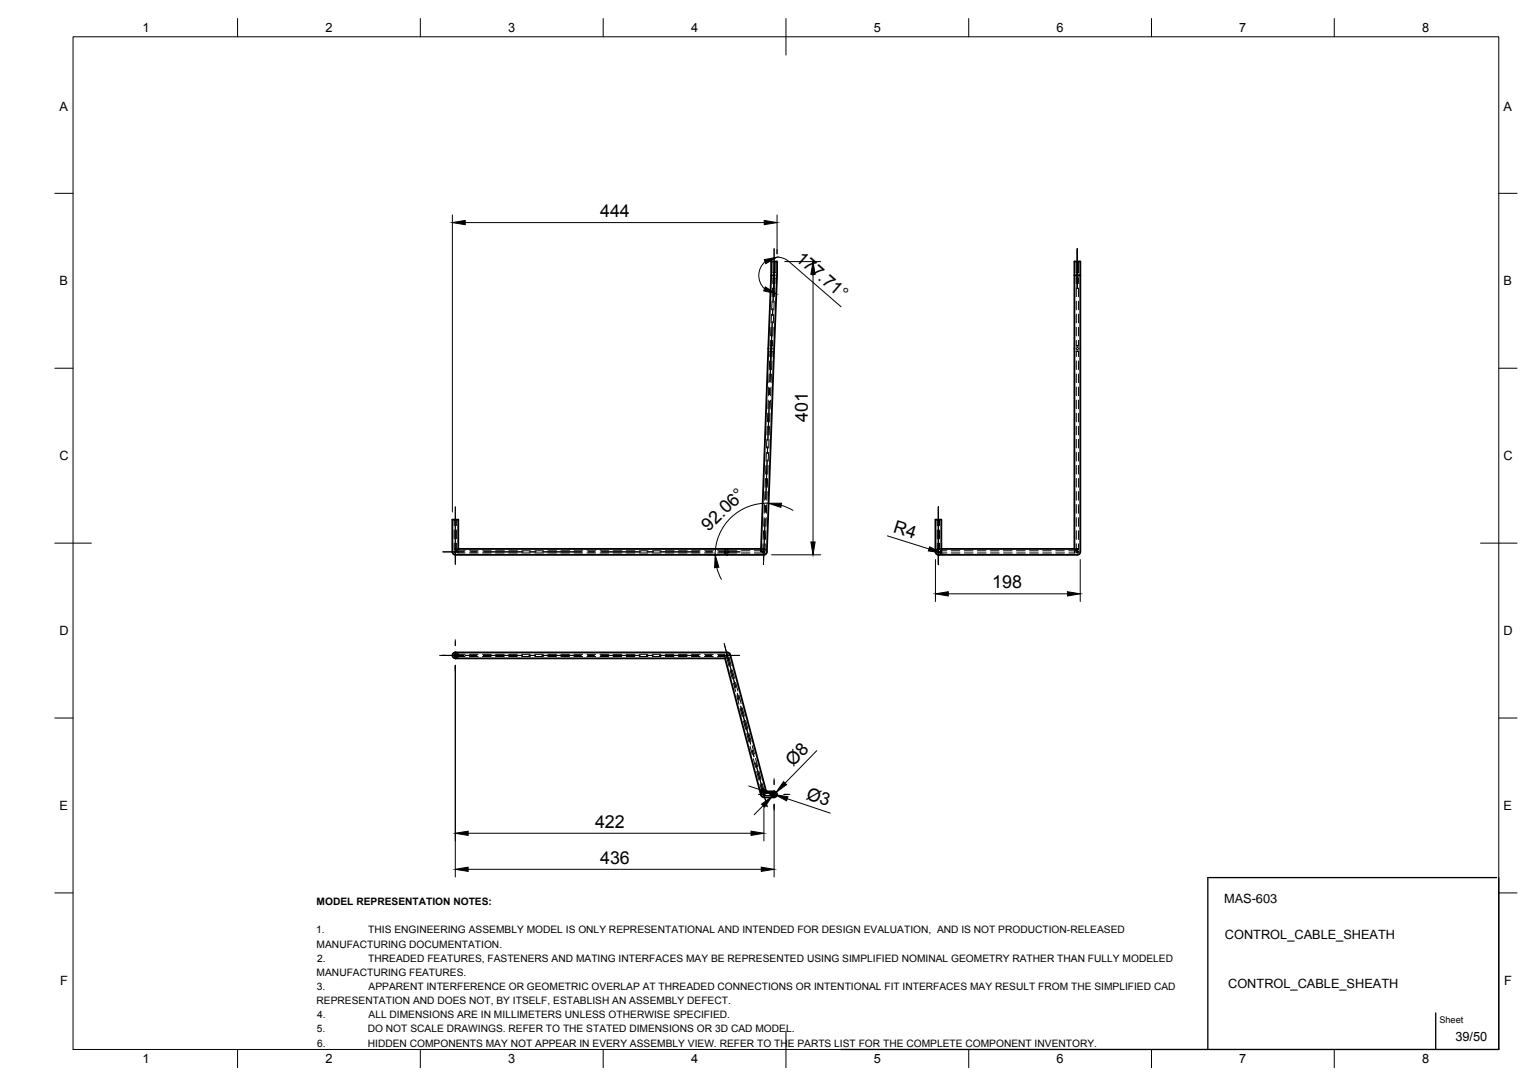
ISO-10303-21;
HEADER;
FILE_DESCRIPTION((''),'2;1');
FILE_NAME('CONTROL_CABLE_SHEATH.step','2026-10-01T22:06:14-07:00',(''),(''),'','','');
FILE_SCHEMA (('AUTOMOTIVE_DESIGN { 1 0 10303 214 3 1 1 }'));
ENDSEC;
DATA;
#10=MECHANICAL_DESIGN_GEOMETRIC_PRESENTATION_REPRESENTATION('',(#1012),#50440);
#21=B_SPLINE_CURVE_WITH_KNOTS('',3,(#47253,#47254,#47255,#47256,#47257,
#47258,#47259,#47260,#47261,#47262),.UNSPECIFIED.,.F.,.F.,(4,2,2,2,4),(0.22845269137107,
0.285543988105223,0.342635284839377,0.399770333790758,0.45690538274214),
 .UNSPECIFIED.) ;
#22=B_SPLINE_CURVE_WITH_KNOTS('',3,(#47263,#47264,#47265,#47266,#47267,
#47268,#47269,#47270,#47271,#47272),.UNSPECIFIED.,.F.,.F.,(4,2,2,2,4),(0.,
0.0571350489513819,0.114270097902764,0.171361394636917,0.22845269137107),
 .UNSPECIFIED.) ;
#23=B_SPLINE_CURVE_WITH_KNOTS('',3,(#47334,#47335,#47336,#47337,#47338,
#47339,#47340,#47341,#47342,#47343,#47344,#47345,#47346,#47347,#47348,#47349,
#47350,#47351),.UNSPECIFIED.,.F.,.F.,(4,2,2,2,2,2,2,2,4),(-0.453190854157869,
-0.399487512163789,-0.342402977588613,-0.285344500479048,-0.228286023369483,
-0.171227546259919,-0.114169069150354,-0.0570845345751771,-0.00338119258109968),
 .UNSPECIFIED.) ;
#24=B_SPLINE_CURVE_WITH_KNOTS('',3,(#47365,#47366,#47367,#47368,#47369,
#47370,#47371,#47372,#47373,#47374,#47375,#47376,#47377,#47378),
 .UNSPECIFIED.,.F.,.F.,(4,2,2,2,2,2,4),(0.577610065542725,0.589037524605606,
0.645581544002731,0.702125563399856,0.758669582796981,0.815213602194107,
0.826641061257004),.UNSPECIFIED.) ;
#25=B_SPLINE_CURVE_WITH_KNOTS('',3,(#47382,#47383,#47384,#47385,#47386,
#47387,#47388,#47389,#47390,#47391,#47392,#47393,#47394,#47395,#47396,#47397,
#47398,#47399),.UNSPECIFIED.,.F.,.F.,(4,2,2,2,2,2,2,2,4),(0.00338117995301888,
0.0570585291380164,0.114117058276033,0.171201519148796,0.228285980021559,
0.285370440894324,0.342454901767089,0.399513430905107,0.453190780090104),
 .UNSPECIFIED.) ;
#26=B_SPLINE_CURVE_WITH_KNOTS('',3,(#47419,#47420,#47421,#47422,#47423,
#47424,#47425,#47426,#47427,#47428,#47429,#47430,#47431,#47432,#47433,#47434,
#47435,#47436),.UNSPECIFIED.,.F.,.F.,(4,2,2,2,2,2,2,2,4),(-0.456905382742139,
-0.399770333790757,-0.342635284839376,-0.285543988105223,-0.228452691371069,
-0.171361394636916,-0.114270097902762,-0.0571350489513811,0.),
 .UNSPECIFIED.) ;
#27=B_SPLINE_CURVE_WITH_KNOTS('',3,(#47442,#47443,#47444,#47445,#47446,
#47447,#47448,#47449,#47450,#47451,#47452,#47453,#47454,#47455),
 .UNSPECIFIED.,.F.,.F.,(4,2,2,2,2,2,4),(0.102836390905491,0.113768884994942,
0.170566995159794,0.227365105324647,0.2841632154895,0.340961325654353,0.351893819743812),
 .UNSPECIFIED.) ;
#68=ORIENTED_CLOSED_SHELL('',*,#28679,.F.) ;
#69=ORIENTED_CLOSED_SHELL('',*,#28680,.F.) ;
#70=ORIENTED_CLOSED_SHELL('',*,#28681,.F.) ;
#71=ORIENTED_CLOSED_SHELL('',*,#28682,.F.) ;
#72=ORIENTED_CLOSED_SHELL('',*,#28684,.F.) ;
#73=ORIENTED_CLOSED_SHELL('',*,#28685,.F.) ;
#74=ORIENTED_CLOSED_SHELL('',*,#28686,.F.) ;
#75=ORIENTED_CLOSED_SHELL('',*,#28687,.F.) ;
#76=ORIENTED_CLOSED_SHELL('',*,#28688,.F.) ;
#80=BREP_WITH_VOIDS('CONTROL_CABLE_SHEATH',#28683,(#68,#69,#70,#71,#72,
#73,#74,#75,#76)) ;
#405=ELLIPSE('',#30976,0.400079928078316,0.4) ;
#406=ELLIPSE('',#30978,0.400079928078316,0.4) ;
#407=ELLIPSE('',#30982,0.400000809214436,0.4) ;
#408=ELLIPSE('',#30983,0.400000809214436,0.4) ;
#409=ELLIPSE('',#30986,0.563115453389195,0.4) ;
#410=ELLIPSE('',#30989,0.505057490139689,0.4) ;
#411=ELLIPSE('',#30992,0.565685424949243,0.4) ;
#412=ELLIPSE('',#30993,0.565685424949243,0.4) ;
#728=SPHERICAL_SURFACE('',#30943,0.15) ;
#729=SPHERICAL_SURFACE('',#30945,0.15) ;
#730=SPHERICAL_SURFACE('',#30947,0.15) ;
#731=SPHERICAL_SURFACE('',#30949,0.4) ;
#732=SPHERICAL_SURFACE('',#30953,0.4) ;
#733=SPHERICAL_SURFACE('',#30954,0.4) ;
#734=SPHERICAL_SURFACE('',#30957,0.4) ;
#735=SPHERICAL_SURFACE('',#30962,0.4) ;
#736=SPHERICAL_SURFACE('',#30965,0.4) ;
#737=SPHERICAL_SURFACE('',#30998,0.4) ;
#738=SPHERICAL_SURFACE('',#30999,0.4) ;
#739=SPHERICAL_SURFACE('',#31000,0.4) ;
#740=SPHERICAL_SURFACE('',#31001,0.4) ;
#741=SPHERICAL_SURFACE('',#31003,0.4) ;
#742=SPHERICAL_SURFACE('',#31009,0.15) ;
#743=SPHERICAL_SURFACE('',#31011,0.4) ;
#744=SPHERICAL_SURFACE('',#31021,0.4) ;
#745=SPHERICAL_SURFACE('',#31022,0.4) ;
#746=SPHERICAL_SURFACE('',#31033,0.4) ;
#747=SPHERICAL_SURFACE('',#31034,0.15) ;
#919=SHAPE_REPRESENTATION_RELATIONSHIP('SRR','None',#50652,#964) ;
#964=ADVANCED_BREP_SHAPE_REPRESENTATION('',(#80),#50421) ;
#1012=STYLED_ITEM('',(#50888),#80) ;
#1377=FACE_BOUND('',#5253,.T.) ;
#1378=FACE_BOUND('',#5261,.T.) ;
#2232=PLANE('',#30979) ;
#2233=PLANE('',#30997) ;
#3420=FACE_OUTER_BOUND('',#5239,.T.) ;
#3421=FACE_OUTER_BOUND('',#5240,.T.) ;
#3422=FACE_OUTER_BOUND('',#5241,.T.) ;
#3423=FACE_OUTER_BOUND('',#5242,.T.) ;
#3424=FACE_OUTER_BOUND('',#5243,.T.) ;
#3425=FACE_OUTER_BOUND('',#5244,.T.) ;
#3426=FACE_OUTER_BOUND('',#5245,.T.) ;
#3427=FACE_OUTER_BOUND('',#5246,.T.) ;
#3428=FACE_OUTER_BOUND('',#5247,.T.) ;
#3429=FACE_OUTER_BOUND('',#5248,.T.) ;
#3430=FACE_OUTER_BOUND('',#5249,.T.) ;
#3431=FACE_OUTER_BOUND('',#5250,.T.) ;
#3432=FACE_OUTER_BOUND('',#5251,.T.) ;
#3433=FACE_OUTER_BOUND('',#5252,.T.) ;
#3434=FACE_OUTER_BOUND('',#5254,.T.) ;
#3435=FACE_OUTER_BOUND('',#5255,.T.) ;
#3436=FACE_OUTER_BOUND('',#5256,.T.) ;
#3437=FACE_OUTER_BOUND('',#5257,.T.) ;
#3438=FACE_OUTER_BOUND('',#5258,.T.) ;
#3439=FACE_OUTER_BOUND('',#5259,.T.) ;
#3440=FACE_OUTER_BOUND('',#5260,.T.) ;
#3441=FACE_OUTER_BOUND('',#5262,.T.) ;
#3442=FACE_OUTER_BOUND('',#5263,.T.) ;
#3443=FACE_OUTER_BOUND('',#5264,.T.) ;
#3444=FACE_OUTER_BOUND('',#5265,.T.) ;
#3445=FACE_OUTER_BOUND('',#5266,.T.) ;
#3446=FACE_OUTER_BOUND('',#5267,.T.) ;
#3447=FACE_OUTER_BOUND('',#5268,.T.) ;
#3448=FACE_OUTER_BOUND('',#5269,.T.) ;
#3449=FACE_OUTER_BOUND('',#5270,.T.) ;
#3450=FACE_OUTER_BOUND('',#5271,.T.) ;
#3451=FACE_OUTER_BOUND('',#5272,.T.) ;
#3452=FACE_OUTER_BOUND('',#5273,.T.) ;
#3453=FACE_OUTER_BOUND('',#5274,.T.) ;
#3454=FACE_OUTER_BOUND('',#5275,.T.) ;
#3455=FACE_OUTER_BOUND('',#5276,.T.) ;
#3456=FACE_OUTER_BOUND('',#5277,.T.) ;
#3457=FACE_OUTER_BOUND('',#5278,.T.) ;
#3458=FACE_OUTER_BOUND('',#5279,.T.) ;
#3459=FACE_OUTER_BOUND('',#5280,.T.) ;
#5239=EDGE_LOOP('',(#24105,#24106)) ;
#5240=EDGE_LOOP('',(#24107,#24108)) ;
#5241=EDGE_LOOP('',(#24109,#24110)) ;
#5242=EDGE_LOOP('',(#24111)) ;
#5243=EDGE_LOOP('',(#24112,#24113,#24114,#24115)) ;
#5244=EDGE_LOOP('',(#24116)) ;
#5245=EDGE_LOOP('',(#24117,#24118)) ;
#5246=EDGE_LOOP('',(#24119,#24120,#24121,#24122)) ;
#5247=EDGE_LOOP('',(#24123,#24124)) ;
#5248=EDGE_LOOP('',(#24125,#24126,#24127)) ;
#5249=EDGE_LOOP('',(#24128,#24129,#24130,#24131,#24132,#24133)) ;
#5250=EDGE_LOOP('',(#24134,#24135,#24136,#24137)) ;
#5251=EDGE_LOOP('',(#24138,#24139,#24140,#24141,#24142,#24143)) ;
#5252=EDGE_LOOP('',(#24144)) ;
#5253=EDGE_LOOP('',(#24145)) ;
#5254=EDGE_LOOP('',(#24146,#24147,#24148,#24149,#24150,#24151,#24152,#24153,
#24154)) ;
#5255=EDGE_LOOP('',(#24155,#24156,#24157,#24158,#24159,#24160,#24161,#24162)) ;
#5256=EDGE_LOOP('',(#24163,#24164,#24165,#24166,#24167,#24168,#24169)) ;
#5257=EDGE_LOOP('',(#24170,#24171,#24172,#24173,#24174,#24175,#24176,#24177)) ;
#5258=EDGE_LOOP('',(#24178,#24179,#24180)) ;
#5259=EDGE_LOOP('',(#24181,#24182,#24183,#24184,#24185,#24186)) ;
#5260=EDGE_LOOP('',(#24187)) ;
#5261=EDGE_LOOP('',(#24188)) ;
#5262=EDGE_LOOP('',(#24189,#24190)) ;
#5263=EDGE_LOOP('',(#24191,#24192,#24193)) ;
#5264=EDGE_LOOP('',(#24194)) ;
#5265=EDGE_LOOP('',(#24195)) ;
#5266=EDGE_LOOP('',(#24196,#24197,#24198)) ;
#5267=EDGE_LOOP('',(#24199,#24200,#24201,#24202,#24203,#24204)) ;
#5268=EDGE_LOOP('',(#24205,#24206)) ;
#5269=EDGE_LOOP('',(#24207,#24208)) ;
#5270=EDGE_LOOP('',(#24209,#24210,#24211)) ;
#5271=EDGE_LOOP('',(#24212,#24213)) ;
#5272=EDGE_LOOP('',(#24214,#24215)) ;
#5273=EDGE_LOOP('',(#24216,#24217,#24218,#24219,#24220,#24221,#24222,#24223)) ;
#5274=EDGE_LOOP('',(#24224,#24225,#24226)) ;
#5275=EDGE_LOOP('',(#24227,#24228,#24229,#24230,#24231)) ;
#5276=EDGE_LOOP('',(#24232,#24233)) ;
#5277=EDGE_LOOP('',(#24234,#24235,#24236,#24237,#24238,#24239,#24240,#24241)) ;
#5278=EDGE_LOOP('',(#24242,#24243)) ;
#5279=EDGE_LOOP('',(#24244,#24245,#24246)) ;
#5280=EDGE_LOOP('',(#24247,#24248)) ;
#7881=LINE('',#47220,#10353) ;
#7882=LINE('',#47252,#10354) ;
#7883=LINE('',#47277,#10355) ;
#7884=LINE('',#47283,#10356) ;
#7885=LINE('',#47294,#10357) ;
#7886=LINE('',#47299,#10358) ;
#7887=LINE('',#47303,#10359) ;
#7888=LINE('',#47309,#10360) ;
#7889=LINE('',#47316,#10361) ;
#7890=LINE('',#47333,#10362) ;
#7891=LINE('',#47403,#10363) ;
#7892=LINE('',#47441,#10364) ;
#10353=VECTOR('',#38012,0.15) ;
#10354=VECTOR('',#38049,0.15) ;
#10355=VECTOR('',#38054,0.15) ;
#10356=VECTOR('',#38061,0.4) ;
#10357=VECTOR('',#38074,0.4) ;
#10358=VECTOR('',#38083,0.4) ;
#10359=VECTOR('',#38088,0.4) ;
#10360=VECTOR('',#38097,0.4) ;
#10361=VECTOR('',#38106,0.4) ;
#10362=VECTOR('',#38131,0.15) ;
#10363=VECTOR('',#38154,0.15) ;
#10364=VECTOR('',#38179,0.15) ;
#11239=CIRCLE('',#30944,0.149999999999999) ;
#11240=CIRCLE('',#30946,0.149999999999999) ;
#11241=CIRCLE('',#30948,0.149999999999999) ;
#11242=CIRCLE('',#30950,0.15) ;
#11243=CIRCLE('',#30952,0.15) ;
#11244=CIRCLE('',#30955,0.4) ;
#11245=CIRCLE('',#30956,0.4) ;
#11246=CIRCLE('',#30958,0.4) ;
#11247=CIRCLE('',#30959,0.4) ;
#11248=CIRCLE('',#30960,0.4) ;
#11249=CIRCLE('',#30961,0.4) ;
#11250=CIRCLE('',#30963,0.4) ;
#11251=CIRCLE('',#30964,0.150000000000006) ;
#11252=CIRCLE('',#30966,0.4) ;
#11253=CIRCLE('',#30967,0.4) ;
#11254=CIRCLE('',#30968,0.4) ;
#11255=CIRCLE('',#30970,0.15) ;
#11256=CIRCLE('',#30972,0.149999999999999) ;
#11257=CIRCLE('',#30973,0.15) ;
#11258=CIRCLE('',#30975,0.4) ;
#11259=CIRCLE('',#30977,0.4) ;
#11260=CIRCLE('',#30981,0.4) ;
#11261=CIRCLE('',#30984,0.4) ;
#11262=CIRCLE('',#30988,0.4) ;
#11263=CIRCLE('',#30991,0.4) ;
#11264=CIRCLE('',#30996,0.4) ;
#11265=CIRCLE('',#31002,0.149999999999999) ;
#11266=CIRCLE('',#31004,0.149999999999999) ;
#11267=CIRCLE('',#31005,0.4) ;
#11268=CIRCLE('',#31006,0.149999999999999) ;
#11269=CIRCLE('',#31010,0.149999999999999) ;
#11270=CIRCLE('',#31012,0.4) ;
#11271=CIRCLE('',#31013,0.149999999999999) ;
#11272=CIRCLE('',#31014,0.149999999999999) ;
#11273=CIRCLE('',#31017,0.4) ;
#11274=CIRCLE('',#31019,0.149999999999999) ;
#11275=CIRCLE('',#31020,0.149999999999999) ;
#11276=CIRCLE('',#31023,0.149999999999999) ;
#11277=CIRCLE('',#31024,0.4) ;
#11278=CIRCLE('',#31025,0.149999999999999) ;
#11279=CIRCLE('',#31026,0.399999999999999) ;
#11280=CIRCLE('',#31028,0.4) ;
#11281=CIRCLE('',#31030,0.149999999999999) ;
#11282=CIRCLE('',#31031,0.149999999999999) ;
#11283=CIRCLE('',#31035,0.149999999999999) ;
#13683=VERTEX_POINT('',#47203) ;
#13684=VERTEX_POINT('',#47204) ;
#13685=VERTEX_POINT('',#47207) ;
#13686=VERTEX_POINT('',#47208) ;
#13687=VERTEX_POINT('',#47211) ;
#13688=VERTEX_POINT('',#47212) ;
#13689=VERTEX_POINT('',#47215) ;
#13690=VERTEX_POINT('',#47218) ;
#13691=VERTEX_POINT('',#47223) ;
#13692=VERTEX_POINT('',#47224) ;
#13693=VERTEX_POINT('',#47228) ;
#13694=VERTEX_POINT('',#47229) ;
#13695=VERTEX_POINT('',#47231) ;
#13696=VERTEX_POINT('',#47233) ;
#13697=VERTEX_POINT('',#47237) ;
#13698=VERTEX_POINT('',#47238) ;
#13699=VERTEX_POINT('',#47242) ;
#13700=VERTEX_POINT('',#47243) ;
#13701=VERTEX_POINT('',#47245) ;
#13702=VERTEX_POINT('',#47249) ;
#13703=VERTEX_POINT('',#47251) ;
#13704=VERTEX_POINT('',#47274) ;
#13705=VERTEX_POINT('',#47276) ;
#13706=VERTEX_POINT('',#47280) ;
#13707=VERTEX_POINT('',#47282) ;
#13708=VERTEX_POINT('',#47284) ;
#13709=VERTEX_POINT('',#47286) ;
#13710=VERTEX_POINT('',#47291) ;
#13711=VERTEX_POINT('',#47293) ;
#13712=VERTEX_POINT('',#47302) ;
#13713=VERTEX_POINT('',#47304) ;
#13714=VERTEX_POINT('',#47310) ;
#13715=VERTEX_POINT('',#47315) ;
#13716=VERTEX_POINT('',#47323) ;
#13717=VERTEX_POINT('',#47326) ;
#13718=VERTEX_POINT('',#47327) ;
#13719=VERTEX_POINT('',#47329) ;
#13720=VERTEX_POINT('',#47354) ;
#13721=VERTEX_POINT('',#47355) ;
#13722=VERTEX_POINT('',#47358) ;
#13723=VERTEX_POINT('',#47359) ;
#13724=VERTEX_POINT('',#47361) ;
#13725=VERTEX_POINT('',#47380) ;
#13726=VERTEX_POINT('',#47381) ;
#13727=VERTEX_POINT('',#47402) ;
#13728=VERTEX_POINT('',#47408) ;
#13729=VERTEX_POINT('',#47409) ;
#13730=VERTEX_POINT('',#47411) ;
#13731=VERTEX_POINT('',#47414) ;
#13732=VERTEX_POINT('',#47417) ;
#13733=VERTEX_POINT('',#47418) ;
#13734=VERTEX_POINT('',#47439) ;
#13735=VERTEX_POINT('',#47460) ;
#13736=VERTEX_POINT('',#47461) ;
#17318=EDGE_CURVE('',#13683,#13684,#11239,.T.) ;
#17319=EDGE_CURVE('',#13685,#13686,#11240,.T.) ;
#17320=EDGE_CURVE('',#13687,#13688,#11241,.T.) ;
#17321=EDGE_CURVE('',#13689,#13689,#11242,.T.) ;
#17322=EDGE_CURVE('',#13690,#13690,#11243,.T.) ;
#17323=EDGE_CURVE('',#13690,#13689,#7881,.T.) ;
#17324=EDGE_CURVE('',#13691,#13692,#11244,.T.) ;
#17325=EDGE_CURVE('',#13692,#13691,#11245,.T.) ;
#17326=EDGE_CURVE('',#13693,#13694,#11246,.T.) ;
#17327=EDGE_CURVE('',#13694,#13695,#11247,.T.) ;
#17328=EDGE_CURVE('',#13695,#13696,#11248,.T.) ;
#17329=EDGE_CURVE('',#13696,#13693,#11249,.T.) ;
#17330=EDGE_CURVE('',#13697,#13698,#11250,.T.) ;
#17331=EDGE_CURVE('',#13697,#13698,#11251,.T.) ;
#17332=EDGE_CURVE('',#13699,#13700,#11252,.T.) ;
#17333=EDGE_CURVE('',#13700,#13701,#11253,.T.) ;
#17334=EDGE_CURVE('',#13701,#13699,#11254,.T.) ;
#17335=EDGE_CURVE('',#13702,#13702,#11255,.T.) ;
#17336=EDGE_CURVE('',#13702,#13703,#7882,.T.) ;
#17337=EDGE_CURVE('',#13703,#13697,#21,.T.) ;
#17338=EDGE_CURVE('',#13698,#13703,#22,.T.) ;
#17339=EDGE_CURVE('',#13704,#13704,#11256,.T.) ;
#17340=EDGE_CURVE('',#13704,#13705,#7883,.T.) ;
#17341=EDGE_CURVE('',#13705,#13705,#11257,.T.) ;
#17342=EDGE_CURVE('',#13706,#13706,#11258,.T.) ;
#17343=EDGE_CURVE('',#13706,#13707,#7884,.T.) ;
#17344=EDGE_CURVE('',#13708,#13707,#405,.T.) ;
#17345=EDGE_CURVE('',#13709,#13708,#11259,.T.) ;
#17346=EDGE_CURVE('',#13707,#13709,#406,.T.) ;
#17347=EDGE_CURVE('',#13710,#13709,#11260,.T.) ;
#17348=EDGE_CURVE('',#13710,#13711,#7885,.T.) ;
#17349=EDGE_CURVE('',#13692,#13711,#407,.T.) ;
#17350=EDGE_CURVE('',#13711,#13691,#408,.T.) ;
#17351=EDGE_CURVE('',#13708,#13710,#11261,.T.) ;
#17352=EDGE_CURVE('',#13711,#13694,#7886,.T.) ;
#17353=EDGE_CURVE('',#13695,#13693,#409,.T.) ;
#17354=EDGE_CURVE('',#13696,#13712,#7887,.T.) ;
#17355=EDGE_CURVE('',#13713,#13712,#11262,.T.) ;
#17356=EDGE_CURVE('',#13712,#13713,#410,.T.) ;
#17357=EDGE_CURVE('',#13712,#13713,#11263,.T.) ;
#17358=EDGE_CURVE('',#13712,#13700,#7888,.T.) ;
#17359=EDGE_CURVE('',#13714,#13699,#411,.T.) ;
#17360=EDGE_CURVE('',#13701,#13714,#412,.T.) ;
#17361=EDGE_CURVE('',#13714,#13715,#7889,.T.) ;
#17362=EDGE_CURVE('',#13715,#13715,#11264,.T.) ;
#17363=EDGE_CURVE('',#13716,#13716,#11265,.T.) ;
#17364=EDGE_CURVE('',#13717,#13718,#11266,.T.) ;
#17365=EDGE_CURVE('',#13717,#13719,#11267,.T.) ;
#17366=EDGE_CURVE('',#13718,#13719,#11268,.T.) ;
#17367=EDGE_CURVE('',#13718,#13716,#7890,.T.) ;
#17368=EDGE_CURVE('',#13717,#13719,#23,.T.) ;
#17369=EDGE_CURVE('',#13720,#13721,#11269,.T.) ;
#17370=EDGE_CURVE('',#13722,#13723,#11270,.T.) ;
#17371=EDGE_CURVE('',#13724,#13723,#11271,.T.) ;
#17372=EDGE_CURVE('',#13722,#13724,#11272,.T.) ;
#17373=EDGE_CURVE('',#13722,#13723,#24,.T.) ;
#17374=EDGE_CURVE('',#13725,#13726,#25,.T.) ;
#17375=EDGE_CURVE('',#13726,#13725,#11273,.T.) ;
#17376=EDGE_CURVE('',#13724,#13727,#7891,.T.) ;
#17377=EDGE_CURVE('',#13727,#13725,#11274,.T.) ;
#17378=EDGE_CURVE('',#13726,#13727,#11275,.T.) ;
#17379=EDGE_CURVE('',#13728,#13729,#11276,.T.) ;
#17380=EDGE_CURVE('',#13728,#13730,#11277,.T.) ;
#17381=EDGE_CURVE('',#13729,#13730,#11278,.T.) ;
#17382=EDGE_CURVE('',#13731,#13729,#11279,.T.) ;
#17383=EDGE_CURVE('',#13732,#13733,#26,.T.) ;
#17384=EDGE_CURVE('',#13732,#13733,#11280,.T.) ;
#17385=EDGE_CURVE('',#13732,#13734,#11281,.T.) ;
#17386=EDGE_CURVE('',#13734,#13729,#7892,.T.) ;
#17387=EDGE_CURVE('',#13730,#13728,#27,.T.) ;
#17388=EDGE_CURVE('',#13734,#13733,#11282,.T.) ;
#17389=EDGE_CURVE('',#13735,#13736,#11283,.T.) ;
#24105=ORIENTED_EDGE('',*,*,#17318,.T.) ;
#24106=ORIENTED_EDGE('',*,*,#17318,.F.) ;
#24107=ORIENTED_EDGE('',*,*,#17319,.T.) ;
#24108=ORIENTED_EDGE('',*,*,#17319,.F.) ;
#24109=ORIENTED_EDGE('',*,*,#17320,.T.) ;
#24110=ORIENTED_EDGE('',*,*,#17320,.F.) ;
#24111=ORIENTED_EDGE('',*,*,#17321,.F.) ;
#24112=ORIENTED_EDGE('',*,*,#17322,.T.) ;
#24113=ORIENTED_EDGE('',*,*,#17323,.T.) ;
#24114=ORIENTED_EDGE('',*,*,#17321,.T.) ;
#24115=ORIENTED_EDGE('',*,*,#17323,.F.) ;
#24116=ORIENTED_EDGE('',*,*,#17322,.F.) ;
#24117=ORIENTED_EDGE('',*,*,#17324,.T.) ;
#24118=ORIENTED_EDGE('',*,*,#17325,.T.) ;
#24119=ORIENTED_EDGE('',*,*,#17326,.T.) ;
#24120=ORIENTED_EDGE('',*,*,#17327,.T.) ;
#24121=ORIENTED_EDGE('',*,*,#17328,.T.) ;
#24122=ORIENTED_EDGE('',*,*,#17329,.T.) ;
#24123=ORIENTED_EDGE('',*,*,#17330,.T.) ;
#24124=ORIENTED_EDGE('',*,*,#17331,.F.) ;
#24125=ORIENTED_EDGE('',*,*,#17332,.T.) ;
#24126=ORIENTED_EDGE('',*,*,#17333,.T.) ;
#24127=ORIENTED_EDGE('',*,*,#17334,.T.) ;
#24128=ORIENTED_EDGE('',*,*,#17335,.F.) ;
#24129=ORIENTED_EDGE('',*,*,#17336,.T.) ;
#24130=ORIENTED_EDGE('',*,*,#17337,.T.) ;
#24131=ORIENTED_EDGE('',*,*,#17331,.T.) ;
#24132=ORIENTED_EDGE('',*,*,#17338,.T.) ;
#24133=ORIENTED_EDGE('',*,*,#17336,.F.) ;
#24134=ORIENTED_EDGE('',*,*,#17339,.T.) ;
#24135=ORIENTED_EDGE('',*,*,#17340,.T.) ;
#24136=ORIENTED_EDGE('',*,*,#17341,.F.) ;
#24137=ORIENTED_EDGE('',*,*,#17340,.F.) ;
#24138=ORIENTED_EDGE('',*,*,#17342,.F.) ;
#24139=ORIENTED_EDGE('',*,*,#17343,.T.) ;
#24140=ORIENTED_EDGE('',*,*,#17344,.F.) ;
#24141=ORIENTED_EDGE('',*,*,#17345,.F.) ;
#24142=ORIENTED_EDGE('',*,*,#17346,.F.) ;
#24143=ORIENTED_EDGE('',*,*,#17343,.F.) ;
#24144=ORIENTED_EDGE('',*,*,#17342,.T.) ;
#24145=ORIENTED_EDGE('',*,*,#17341,.T.) ;
#24146=ORIENTED_EDGE('',*,*,#17344,.T.) ;
#24147=ORIENTED_EDGE('',*,*,#17346,.T.) ;
#24148=ORIENTED_EDGE('',*,*,#17347,.F.) ;
#24149=ORIENTED_EDGE('',*,*,#17348,.T.) ;
#24150=ORIENTED_EDGE('',*,*,#17349,.F.) ;
#24151=ORIENTED_EDGE('',*,*,#17324,.F.) ;
#24152=ORIENTED_EDGE('',*,*,#17350,.F.) ;
#24153=ORIENTED_EDGE('',*,*,#17348,.F.) ;
#24154=ORIENTED_EDGE('',*,*,#17351,.F.) ;
#24155=ORIENTED_EDGE('',*,*,#17349,.T.) ;
#24156=ORIENTED_EDGE('',*,*,#17352,.T.) ;
#24157=ORIENTED_EDGE('',*,*,#17326,.F.) ;
#24158=ORIENTED_EDGE('',*,*,#17353,.F.) ;
#24159=ORIENTED_EDGE('',*,*,#17327,.F.) ;
#24160=ORIENTED_EDGE('',*,*,#17352,.F.) ;
#24161=ORIENTED_EDGE('',*,*,#17350,.T.) ;
#24162=ORIENTED_EDGE('',*,*,#17325,.F.) ;
#24163=ORIENTED_EDGE('',*,*,#17353,.T.) ;
#24164=ORIENTED_EDGE('',*,*,#17329,.F.) ;
#24165=ORIENTED_EDGE('',*,*,#17354,.T.) ;
#24166=ORIENTED_EDGE('',*,*,#17355,.F.) ;
#24167=ORIENTED_EDGE('',*,*,#17356,.F.) ;
#24168=ORIENTED_EDGE('',*,*,#17354,.F.) ;
#24169=ORIENTED_EDGE('',*,*,#17328,.F.) ;
#24170=ORIENTED_EDGE('',*,*,#17356,.T.) ;
#24171=ORIENTED_EDGE('',*,*,#17357,.F.) ;
#24172=ORIENTED_EDGE('',*,*,#17358,.T.) ;
#24173=ORIENTED_EDGE('',*,*,#17332,.F.) ;
#24174=ORIENTED_EDGE('',*,*,#17359,.F.) ;
#24175=ORIENTED_EDGE('',*,*,#17360,.F.) ;
#24176=ORIENTED_EDGE('',*,*,#17333,.F.) ;
#24177=ORIENTED_EDGE('',*,*,#17358,.F.) ;
#24178=ORIENTED_EDGE('',*,*,#17338,.F.) ;
#24179=ORIENTED_EDGE('',*,*,#17330,.F.) ;
#24180=ORIENTED_EDGE('',*,*,#17337,.F.) ;
#24181=ORIENTED_EDGE('',*,*,#17360,.T.) ;
#24182=ORIENTED_EDGE('',*,*,#17361,.T.) ;
#24183=ORIENTED_EDGE('',*,*,#17362,.F.) ;
#24184=ORIENTED_EDGE('',*,*,#17361,.F.) ;
#24185=ORIENTED_EDGE('',*,*,#17359,.T.) ;
#24186=ORIENTED_EDGE('',*,*,#17334,.F.) ;
#24187=ORIENTED_EDGE('',*,*,#17362,.T.) ;
#24188=ORIENTED_EDGE('',*,*,#17335,.T.) ;
#24189=ORIENTED_EDGE('',*,*,#17357,.T.) ;
#24190=ORIENTED_EDGE('',*,*,#17355,.T.) ;
#24191=ORIENTED_EDGE('',*,*,#17351,.T.) ;
#24192=ORIENTED_EDGE('',*,*,#17347,.T.) ;
#24193=ORIENTED_EDGE('',*,*,#17345,.T.) ;
#24194=ORIENTED_EDGE('',*,*,#17339,.F.) ;
#24195=ORIENTED_EDGE('',*,*,#17363,.F.) ;
#24196=ORIENTED_EDGE('',*,*,#17364,.F.) ;
#24197=ORIENTED_EDGE('',*,*,#17365,.T.) ;
#24198=ORIENTED_EDGE('',*,*,#17366,.F.) ;
#24199=ORIENTED_EDGE('',*,*,#17364,.T.) ;
#24200=ORIENTED_EDGE('',*,*,#17367,.T.) ;
#24201=ORIENTED_EDGE('',*,*,#17363,.T.) ;
#24202=ORIENTED_EDGE('',*,*,#17367,.F.) ;
#24203=ORIENTED_EDGE('',*,*,#17366,.T.) ;
#24204=ORIENTED_EDGE('',*,*,#17368,.F.) ;
#24205=ORIENTED_EDGE('',*,*,#17368,.T.) ;
#24206=ORIENTED_EDGE('',*,*,#17365,.F.) ;
#24207=ORIENTED_EDGE('',*,*,#17369,.T.) ;
#24208=ORIENTED_EDGE('',*,*,#17369,.F.) ;
#24209=ORIENTED_EDGE('',*,*,#17370,.T.) ;
#24210=ORIENTED_EDGE('',*,*,#17371,.F.) ;
#24211=ORIENTED_EDGE('',*,*,#17372,.F.) ;
#24212=ORIENTED_EDGE('',*,*,#17373,.T.) ;
#24213=ORIENTED_EDGE('',*,*,#17370,.F.) ;
#24214=ORIENTED_EDGE('',*,*,#17374,.F.) ;
#24215=ORIENTED_EDGE('',*,*,#17375,.F.) ;
#24216=ORIENTED_EDGE('',*,*,#17372,.T.) ;
#24217=ORIENTED_EDGE('',*,*,#17376,.T.) ;
#24218=ORIENTED_EDGE('',*,*,#17377,.T.) ;
#24219=ORIENTED_EDGE('',*,*,#17374,.T.) ;
#24220=ORIENTED_EDGE('',*,*,#17378,.T.) ;
#24221=ORIENTED_EDGE('',*,*,#17376,.F.) ;
#24222=ORIENTED_EDGE('',*,*,#17371,.T.) ;
#24223=ORIENTED_EDGE('',*,*,#17373,.F.) ;
#24224=ORIENTED_EDGE('',*,*,#17375,.T.) ;
#24225=ORIENTED_EDGE('',*,*,#17377,.F.) ;
#24226=ORIENTED_EDGE('',*,*,#17378,.F.) ;
#24227=ORIENTED_EDGE('',*,*,#17379,.F.) ;
#24228=ORIENTED_EDGE('',*,*,#17380,.T.) ;
#24229=ORIENTED_EDGE('',*,*,#17381,.F.) ;
#24230=ORIENTED_EDGE('',*,*,#17382,.F.) ;
#24231=ORIENTED_EDGE('',*,*,#17382,.T.) ;
#24232=ORIENTED_EDGE('',*,*,#17383,.T.) ;
#24233=ORIENTED_EDGE('',*,*,#17384,.F.) ;
#24234=ORIENTED_EDGE('',*,*,#17385,.T.) ;
#24235=ORIENTED_EDGE('',*,*,#17386,.T.) ;
#24236=ORIENTED_EDGE('',*,*,#17381,.T.) ;
#24237=ORIENTED_EDGE('',*,*,#17387,.T.) ;
#24238=ORIENTED_EDGE('',*,*,#17379,.T.) ;
#24239=ORIENTED_EDGE('',*,*,#17386,.F.) ;
#24240=ORIENTED_EDGE('',*,*,#17388,.T.) ;
#24241=ORIENTED_EDGE('',*,*,#17383,.F.) ;
#24242=ORIENTED_EDGE('',*,*,#17387,.F.) ;
#24243=ORIENTED_EDGE('',*,*,#17380,.F.) ;
#24244=ORIENTED_EDGE('',*,*,#17385,.F.) ;
#24245=ORIENTED_EDGE('',*,*,#17384,.T.) ;
#24246=ORIENTED_EDGE('',*,*,#17388,.F.) ;
#24247=ORIENTED_EDGE('',*,*,#17389,.T.) ;
#24248=ORIENTED_EDGE('',*,*,#17389,.F.) ;
#26872=CYLINDRICAL_SURFACE('',#30951,0.15) ;
#26873=CYLINDRICAL_SURFACE('',#30969,0.15) ;
#26874=CYLINDRICAL_SURFACE('',#30971,0.15) ;
#26875=CYLINDRICAL_SURFACE('',#30974,0.4) ;
#26876=CYLINDRICAL_SURFACE('',#30980,0.4) ;
#26877=CYLINDRICAL_SURFACE('',#30985,0.4) ;
#26878=CYLINDRICAL_SURFACE('',#30987,0.4) ;
#26879=CYLINDRICAL_SURFACE('',#30990,0.4) ;
#26880=CYLINDRICAL_SURFACE('',#30994,0.4) ;
#26881=CYLINDRICAL_SURFACE('',#30995,0.4) ;
#26882=CYLINDRICAL_SURFACE('',#31007,0.15) ;
#26883=CYLINDRICAL_SURFACE('',#31008,0.4) ;
#26884=CYLINDRICAL_SURFACE('',#31015,0.4) ;
#26885=CYLINDRICAL_SURFACE('',#31016,0.4) ;
#26886=CYLINDRICAL_SURFACE('',#31018,0.15) ;
#26887=CYLINDRICAL_SURFACE('',#31027,0.4) ;
#26888=CYLINDRICAL_SURFACE('',#31029,0.15) ;
#26889=CYLINDRICAL_SURFACE('',#31032,0.4) ;
#28155=ADVANCED_FACE('',(#3420),#728,.F.) ;
#28156=ADVANCED_FACE('',(#3421),#729,.F.) ;
#28157=ADVANCED_FACE('',(#3422),#730,.F.) ;
#28158=ADVANCED_FACE('',(#3423),#731,.T.) ;
#28159=ADVANCED_FACE('',(#3424),#26872,.F.) ;
#28160=ADVANCED_FACE('',(#3425),#732,.T.) ;
#28161=ADVANCED_FACE('',(#3426),#733,.T.) ;
#28162=ADVANCED_FACE('',(#3427),#734,.T.) ;
#28163=ADVANCED_FACE('',(#3428),#735,.T.) ;
#28164=ADVANCED_FACE('',(#3429),#736,.T.) ;
#28165=ADVANCED_FACE('',(#3430),#26873,.F.) ;
#28166=ADVANCED_FACE('',(#3431),#26874,.F.) ;
#28167=ADVANCED_FACE('',(#3432),#26875,.T.) ;
#28168=ADVANCED_FACE('',(#3433,#1377),#2232,.T.) ;
#28169=ADVANCED_FACE('',(#3434),#26876,.T.) ;
#28170=ADVANCED_FACE('',(#3435),#26877,.T.) ;
#28171=ADVANCED_FACE('',(#3436),#26878,.T.) ;
#28172=ADVANCED_FACE('',(#3437),#26879,.T.) ;
#28173=ADVANCED_FACE('',(#3438),#26880,.T.) ;
#28174=ADVANCED_FACE('',(#3439),#26881,.T.) ;
#28175=ADVANCED_FACE('',(#3440,#1378),#2233,.T.) ;
#28176=ADVANCED_FACE('',(#3441),#737,.T.) ;
#28177=ADVANCED_FACE('',(#3442),#738,.T.) ;
#28178=ADVANCED_FACE('',(#3443),#739,.T.) ;
#28179=ADVANCED_FACE('',(#3444),#740,.T.) ;
#28180=ADVANCED_FACE('',(#3445),#741,.T.) ;
#28181=ADVANCED_FACE('',(#3446),#26882,.F.) ;
#28182=ADVANCED_FACE('',(#3447),#26883,.T.) ;
#28183=ADVANCED_FACE('',(#3448),#742,.F.) ;
#28184=ADVANCED_FACE('',(#3449),#743,.T.) ;
#28185=ADVANCED_FACE('',(#3450),#26884,.T.) ;
#28186=ADVANCED_FACE('',(#3451),#26885,.T.) ;
#28187=ADVANCED_FACE('',(#3452),#26886,.F.) ;
#28188=ADVANCED_FACE('',(#3453),#744,.T.) ;
#28189=ADVANCED_FACE('',(#3454),#745,.T.) ;
#28190=ADVANCED_FACE('',(#3455),#26887,.T.) ;
#28191=ADVANCED_FACE('',(#3456),#26888,.F.) ;
#28192=ADVANCED_FACE('',(#3457),#26889,.T.) ;
#28193=ADVANCED_FACE('',(#3458),#746,.T.) ;
#28194=ADVANCED_FACE('',(#3459),#747,.F.) ;
#28679=CLOSED_SHELL('',(#28155)) ;
#28680=CLOSED_SHELL('',(#28156)) ;
#28681=CLOSED_SHELL('',(#28157)) ;
#28682=CLOSED_SHELL('',(#28158,#28159,#28160)) ;
#28683=CLOSED_SHELL('',(#28161,#28162,#28163,#28164,#28165,#28166,#28167,
#28168,#28169,#28170,#28171,#28172,#28173,#28174,#28175,#28176,#28177,#28178)) ;
#28684=CLOSED_SHELL('',(#28179,#28180,#28181,#28182)) ;
#28685=CLOSED_SHELL('',(#28183)) ;
#28686=CLOSED_SHELL('',(#28184,#28185,#28186,#28187,#28188)) ;
#28687=CLOSED_SHELL('',(#28189,#28190,#28191,#28192,#28193)) ;
#28688=CLOSED_SHELL('',(#28194)) ;
#30942=AXIS2_PLACEMENT_3D('',#47201,#37990,#37991) ;
#30943=AXIS2_PLACEMENT_3D('',#47202,#37992,#37993) ;
#30944=AXIS2_PLACEMENT_3D('',#47205,#37994,#37995) ;
#30945=AXIS2_PLACEMENT_3D('',#47206,#37996,#37997) ;
#30946=AXIS2_PLACEMENT_3D('',#47209,#37998,#37999) ;
#30947=AXIS2_PLACEMENT_3D('',#47210,#38000,#38001) ;
#30948=AXIS2_PLACEMENT_3D('',#47213,#38002,#38003) ;
#30949=AXIS2_PLACEMENT_3D('',#47214,#38004,#38005) ;
#30950=AXIS2_PLACEMENT_3D('',#47216,#38006,#38007) ;
#30951=AXIS2_PLACEMENT_3D('',#47217,#38008,#38009) ;
#30952=AXIS2_PLACEMENT_3D('',#47219,#38010,#38011) ;
#30953=AXIS2_PLACEMENT_3D('',#47221,#38013,#38014) ;
#30954=AXIS2_PLACEMENT_3D('',#47222,#38015,#38016) ;
#30955=AXIS2_PLACEMENT_3D('',#47225,#38017,#38018) ;
#30956=AXIS2_PLACEMENT_3D('',#47226,#38019,#38020) ;
#30957=AXIS2_PLACEMENT_3D('',#47227,#38021,#38022) ;
#30958=AXIS2_PLACEMENT_3D('',#47230,#38023,#38024) ;
#30959=AXIS2_PLACEMENT_3D('',#47232,#38025,#38026) ;
#30960=AXIS2_PLACEMENT_3D('',#47234,#38027,#38028) ;
#30961=AXIS2_PLACEMENT_3D('',#47235,#38029,#38030) ;
#30962=AXIS2_PLACEMENT_3D('',#47236,#38031,#38032) ;
#30963=AXIS2_PLACEMENT_3D('',#47239,#38033,#38034) ;
#30964=AXIS2_PLACEMENT_3D('',#47240,#38035,#38036) ;
#30965=AXIS2_PLACEMENT_3D('',#47241,#38037,#38038) ;
#30966=AXIS2_PLACEMENT_3D('',#47244,#38039,#38040) ;
#30967=AXIS2_PLACEMENT_3D('',#47246,#38041,#38042) ;
#30968=AXIS2_PLACEMENT_3D('',#47247,#38043,#38044) ;
#30969=AXIS2_PLACEMENT_3D('',#47248,#38045,#38046) ;
#30970=AXIS2_PLACEMENT_3D('',#47250,#38047,#38048) ;
#30971=AXIS2_PLACEMENT_3D('',#47273,#38050,#38051) ;
#30972=AXIS2_PLACEMENT_3D('',#47275,#38052,#38053) ;
#30973=AXIS2_PLACEMENT_3D('',#47278,#38055,#38056) ;
#30974=AXIS2_PLACEMENT_3D('',#47279,#38057,#38058) ;
#30975=AXIS2_PLACEMENT_3D('',#47281,#38059,#38060) ;
#30976=AXIS2_PLACEMENT_3D('',#47285,#38062,#38063) ;
#30977=AXIS2_PLACEMENT_3D('',#47287,#38064,#38065) ;
#30978=AXIS2_PLACEMENT_3D('',#47288,#38066,#38067) ;
#30979=AXIS2_PLACEMENT_3D('',#47289,#38068,#38069) ;
#30980=AXIS2_PLACEMENT_3D('',#47290,#38070,#38071) ;
#30981=AXIS2_PLACEMENT_3D('',#47292,#38072,#38073) ;
#30982=AXIS2_PLACEMENT_3D('',#47295,#38075,#38076) ;
#30983=AXIS2_PLACEMENT_3D('',#47296,#38077,#38078) ;
#30984=AXIS2_PLACEMENT_3D('',#47297,#38079,#38080) ;
#30985=AXIS2_PLACEMENT_3D('',#47298,#38081,#38082) ;
#30986=AXIS2_PLACEMENT_3D('',#47300,#38084,#38085) ;
#30987=AXIS2_PLACEMENT_3D('',#47301,#38086,#38087) ;
#30988=AXIS2_PLACEMENT_3D('',#47305,#38089,#38090) ;
#30989=AXIS2_PLACEMENT_3D('',#47306,#38091,#38092) ;
#30990=AXIS2_PLACEMENT_3D('',#47307,#38093,#38094) ;
#30991=AXIS2_PLACEMENT_3D('',#47308,#38095,#38096) ;
#30992=AXIS2_PLACEMENT_3D('',#47311,#38098,#38099) ;
#30993=AXIS2_PLACEMENT_3D('',#47312,#38100,#38101) ;
#30994=AXIS2_PLACEMENT_3D('',#47313,#38102,#38103) ;
#30995=AXIS2_PLACEMENT_3D('',#47314,#38104,#38105) ;
#30996=AXIS2_PLACEMENT_3D('',#47317,#38107,#38108) ;
#30997=AXIS2_PLACEMENT_3D('',#47318,#38109,#38110) ;
#30998=AXIS2_PLACEMENT_3D('',#47319,#38111,#38112) ;
#30999=AXIS2_PLACEMENT_3D('',#47320,#38113,#38114) ;
#31000=AXIS2_PLACEMENT_3D('',#47321,#38115,#38116) ;
#31001=AXIS2_PLACEMENT_3D('',#47322,#38117,#38118) ;
#31002=AXIS2_PLACEMENT_3D('',#47324,#38119,#38120) ;
#31003=AXIS2_PLACEMENT_3D('',#47325,#38121,#38122) ;
#31004=AXIS2_PLACEMENT_3D('',#47328,#38123,#38124) ;
#31005=AXIS2_PLACEMENT_3D('',#47330,#38125,#38126) ;
#31006=AXIS2_PLACEMENT_3D('',#47331,#38127,#38128) ;
#31007=AXIS2_PLACEMENT_3D('',#47332,#38129,#38130) ;
#31008=AXIS2_PLACEMENT_3D('',#47352,#38132,#38133) ;
#31009=AXIS2_PLACEMENT_3D('',#47353,#38134,#38135) ;
#31010=AXIS2_PLACEMENT_3D('',#47356,#38136,#38137) ;
#31011=AXIS2_PLACEMENT_3D('',#47357,#38138,#38139) ;
#31012=AXIS2_PLACEMENT_3D('',#47360,#38140,#38141) ;
#31013=AXIS2_PLACEMENT_3D('',#47362,#38142,#38143) ;
#31014=AXIS2_PLACEMENT_3D('',#47363,#38144,#38145) ;
#31015=AXIS2_PLACEMENT_3D('',#47364,#38146,#38147) ;
#31016=AXIS2_PLACEMENT_3D('',#47379,#38148,#38149) ;
#31017=AXIS2_PLACEMENT_3D('',#47400,#38150,#38151) ;
#31018=AXIS2_PLACEMENT_3D('',#47401,#38152,#38153) ;
#31019=AXIS2_PLACEMENT_3D('',#47404,#38155,#38156) ;
#31020=AXIS2_PLACEMENT_3D('',#47405,#38157,#38158) ;
#31021=AXIS2_PLACEMENT_3D('',#47406,#38159,#38160) ;
#31022=AXIS2_PLACEMENT_3D('',#47407,#38161,#38162) ;
#31023=AXIS2_PLACEMENT_3D('',#47410,#38163,#38164) ;
#31024=AXIS2_PLACEMENT_3D('',#47412,#38165,#38166) ;
#31025=AXIS2_PLACEMENT_3D('',#47413,#38167,#38168) ;
#31026=AXIS2_PLACEMENT_3D('',#47415,#38169,#38170) ;
#31027=AXIS2_PLACEMENT_3D('',#47416,#38171,#38172) ;
#31028=AXIS2_PLACEMENT_3D('',#47437,#38173,#38174) ;
#31029=AXIS2_PLACEMENT_3D('',#47438,#38175,#38176) ;
#31030=AXIS2_PLACEMENT_3D('',#47440,#38177,#38178) ;
#31031=AXIS2_PLACEMENT_3D('',#47456,#38180,#38181) ;
#31032=AXIS2_PLACEMENT_3D('',#47457,#38182,#38183) ;
#31033=AXIS2_PLACEMENT_3D('',#47458,#38184,#38185) ;
#31034=AXIS2_PLACEMENT_3D('',#47459,#38186,#38187) ;
#31035=AXIS2_PLACEMENT_3D('',#47462,#38188,#38189) ;
#37990=DIRECTION('axis',(0.,0.,1.)) ;
#37991=DIRECTION('refdir',(1.,0.,0.)) ;
#37992=DIRECTION('center_axis',(0.,0.,1.)) ;
#37993=DIRECTION('ref_axis',(1.,0.,0.)) ;
#37994=DIRECTION('center_axis',(0.,1.,0.)) ;
#37995=DIRECTION('ref_axis',(-1.,0.,0.)) ;
#37996=DIRECTION('center_axis',(0.,0.,1.)) ;
#37997=DIRECTION('ref_axis',(1.,0.,0.)) ;
#37998=DIRECTION('center_axis',(-1.22464679914737E-16,1.,0.)) ;
#37999=DIRECTION('ref_axis',(-1.,-1.22464679914737E-16,0.)) ;
#38000=DIRECTION('center_axis',(0.,0.,1.)) ;
#38001=DIRECTION('ref_axis',(1.,0.,0.)) ;
#38002=DIRECTION('center_axis',(-1.22464679914737E-16,1.,0.)) ;
#38003=DIRECTION('ref_axis',(-1.,-1.22464679914737E-16,0.)) ;
#38004=DIRECTION('center_axis',(0.,-1.22927471708385E-18,1.)) ;
#38005=DIRECTION('ref_axis',(-0.99979846524302,-0.0200755796355278,0.)) ;
#38006=DIRECTION('center_axis',(0.999200958721789,0.,-0.0399680383488722)) ;
#38007=DIRECTION('ref_axis',(0.0399680383488744,0.,0.999200958721789)) ;
#38008=DIRECTION('center_axis',(0.999200958721789,0.,-0.0399680383488722)) ;
#38009=DIRECTION('ref_axis',(0.0399680383488722,0.,0.999200958721789)) ;
#38010=DIRECTION('center_axis',(-0.999200958721789,0.,0.0399680383488722)) ;
#38011=DIRECTION('ref_axis',(0.0399680383488744,0.,0.999200958721789)) ;
#38012=DIRECTION('',(0.999200958721789,0.,-0.0399680383488722)) ;
#38013=DIRECTION('center_axis',(0.,0.,1.)) ;
#38014=DIRECTION('ref_axis',(1.,0.,0.)) ;
#38015=DIRECTION('center_axis',(0.,0.,1.)) ;
#38016=DIRECTION('ref_axis',(1.,0.,0.)) ;
#38017=DIRECTION('center_axis',(-0.999200958721789,0.,0.0399680383488714)) ;
#38018=DIRECTION('ref_axis',(0.0399680383488714,0.,0.999200958721789)) ;
#38019=DIRECTION('center_axis',(0.999353662725428,0.,-0.035947973479332)) ;
#38020=DIRECTION('ref_axis',(0.035947973479332,0.,0.999353662725428)) ;
#38021=DIRECTION('center_axis',(0.,-8.29277425593329E-18,1.)) ;
#38022=DIRECTION('ref_axis',(-0.990786741964199,-0.135431281275663,0.)) ;
#38023=DIRECTION('center_axis',(-0.999353662725428,0.,0.035947973479332)) ;
#38024=DIRECTION('ref_axis',(0.035947973479332,0.,0.999353662725428)) ;
#38025=DIRECTION('center_axis',(-0.999353662725428,0.,0.035947973479332)) ;
#38026=DIRECTION('ref_axis',(0.035947973479332,0.,0.999353662725428)) ;
#38027=DIRECTION('center_axis',(0.,-0.967074537262646,-0.254493299279644)) ;
#38028=DIRECTION('ref_axis',(1.,0.,0.)) ;
#38029=DIRECTION('center_axis',(0.,-0.967074537262646,-0.254493299279644)) ;
#38030=DIRECTION('ref_axis',(1.,0.,0.)) ;
#38031=DIRECTION('center_axis',(0.,0.,1.)) ;
#38032=DIRECTION('ref_axis',(1.,0.,0.)) ;
#38033=DIRECTION('center_axis',(0.,0.,1.)) ;
#38034=DIRECTION('ref_axis',(1.,0.,0.)) ;
#38035=DIRECTION('center_axis',(-1.,0.,0.)) ;
#38036=DIRECTION('ref_axis',(0.,0.,1.)) ;
#38037=DIRECTION('center_axis',(0.577350269189626,0.577350269189626,0.577350269189626)) ;
#38038=DIRECTION('ref_axis',(-0.707106781186548,0.,0.707106781186548)) ;
#38039=DIRECTION('center_axis',(0.,0.,1.)) ;
#38040=DIRECTION('ref_axis',(1.,0.,0.)) ;
#38041=DIRECTION('center_axis',(0.,0.,1.)) ;
#38042=DIRECTION('ref_axis',(1.,0.,0.)) ;
#38043=DIRECTION('center_axis',(-1.,0.,0.)) ;
#38044=DIRECTION('ref_axis',(0.,0.,1.)) ;
#38045=DIRECTION('center_axis',(-1.,0.,0.)) ;
#38046=DIRECTION('ref_axis',(0.,0.,1.)) ;
#38047=DIRECTION('center_axis',(-1.,0.,0.)) ;
#38048=DIRECTION('ref_axis',(0.,0.,1.)) ;
#38049=DIRECTION('',(-1.,0.,0.)) ;
#38050=DIRECTION('center_axis',(1.,0.,0.)) ;
#38051=DIRECTION('ref_axis',(0.,0.,-1.)) ;
#38052=DIRECTION('center_axis',(-1.,0.,0.)) ;
#38053=DIRECTION('ref_axis',(0.,0.,-1.)) ;
#38054=DIRECTION('',(1.,0.,0.)) ;
#38055=DIRECTION('center_axis',(-1.,0.,0.)) ;
#38056=DIRECTION('ref_axis',(0.,0.,-1.)) ;
#38057=DIRECTION('center_axis',(1.,0.,0.)) ;
#38058=DIRECTION('ref_axis',(0.,0.,-1.)) ;
#38059=DIRECTION('center_axis',(1.,0.,0.)) ;
#38060=DIRECTION('ref_axis',(0.,0.,-1.)) ;
#38061=DIRECTION('',(-1.,0.,0.)) ;
#38062=DIRECTION('center_axis',(-0.999800219724343,0.,0.0199880123863293)) ;
#38063=DIRECTION('ref_axis',(-0.0199880123863293,0.,-0.999800219724343)) ;
#38064=DIRECTION('center_axis',(-1.,0.,0.)) ;
#38065=DIRECTION('ref_axis',(0.,0.,-1.)) ;
#38066=DIRECTION('center_axis',(-0.999800219724343,0.,0.0199880123863293)) ;
#38067=DIRECTION('ref_axis',(-0.0199880123863293,0.,-0.999800219724343)) ;
#38068=DIRECTION('center_axis',(1.,0.,0.)) ;
#38069=DIRECTION('ref_axis',(0.,0.,-1.)) ;
#38070=DIRECTION('center_axis',(0.999200958721789,0.,-0.0399680383488714)) ;
#38071=DIRECTION('ref_axis',(0.0399680383488714,0.,0.999200958721789)) ;
#38072=DIRECTION('center_axis',(0.999200958721789,0.,-0.0399680383488714)) ;
#38073=DIRECTION('ref_axis',(0.0399680383488714,0.,0.999200958721789)) ;
#38074=DIRECTION('',(-0.999200958721789,0.,0.0399680383488714)) ;
#38075=DIRECTION('center_axis',(-0.999279332296661,0.,0.0379580827326481)) ;
#38076=DIRECTION('ref_axis',(0.0379580827326481,0.,0.999279332296661)) ;
#38077=DIRECTION('center_axis',(-0.999279332296661,0.,0.0379580827326481)) ;
#38078=DIRECTION('ref_axis',(0.0379580827326481,0.,0.999279332296661)) ;
#38079=DIRECTION('center_axis',(0.999200958721789,0.,-0.0399680383488714)) ;
#38080=DIRECTION('ref_axis',(0.0399680383488714,0.,0.999200958721789)) ;
#38081=DIRECTION('center_axis',(0.999353662725428,0.,-0.035947973479332)) ;
#38082=DIRECTION('ref_axis',(0.035947973479332,0.,0.999353662725428)) ;
#38083=DIRECTION('',(-0.999353662725428,0.,0.035947973479332)) ;
#38084=DIRECTION('center_axis',(-0.703439363602225,0.680718270639751,0.20443996124076)) ;
#38085=DIRECTION('ref_axis',(0.709904500032622,0.686974583149487,0.155246651944643)) ;
#38086=DIRECTION('center_axis',(0.,-0.967074537262646,-0.254493299279644)) ;
#38087=DIRECTION('ref_axis',(1.,0.,0.)) ;
#38088=DIRECTION('',(0.,0.967074537262646,0.254493299279644)) ;
#38089=DIRECTION('center_axis',(0.,0.967074537262646,0.254493299279644)) ;
#38090=DIRECTION('ref_axis',(1.,0.,0.)) ;
#38091=DIRECTION('center_axis',(0.,0.610535298209836,0.791989046414044)) ;
#38092=DIRECTION('ref_axis',(0.,-0.791989046414044,0.610535298209836)) ;
#38093=DIRECTION('center_axis',(0.,0.,-1.)) ;
#38094=DIRECTION('ref_axis',(1.,0.,0.)) ;
#38095=DIRECTION('center_axis',(0.,0.,-1.)) ;
#38096=DIRECTION('ref_axis',(1.,0.,0.)) ;
#38097=DIRECTION('',(0.,0.,1.)) ;
#38098=DIRECTION('center_axis',(0.707106781186554,0.,0.707106781186541)) ;
#38099=DIRECTION('ref_axis',(0.707106781186541,0.,-0.707106781186554)) ;
#38100=DIRECTION('center_axis',(0.707106781186554,0.,0.707106781186541)) ;
#38101=DIRECTION('ref_axis',(0.707106781186541,0.,-0.707106781186554)) ;
#38102=DIRECTION('center_axis',(0.,0.,-1.)) ;
#38103=DIRECTION('ref_axis',(1.,0.,0.)) ;
#38104=DIRECTION('center_axis',(-1.,0.,0.)) ;
#38105=DIRECTION('ref_axis',(0.,0.,1.)) ;
#38106=DIRECTION('',(1.,0.,0.)) ;
#38107=DIRECTION('center_axis',(1.,0.,0.)) ;
#38108=DIRECTION('ref_axis',(0.,0.,1.)) ;
#38109=DIRECTION('center_axis',(1.,0.,0.)) ;
#38110=DIRECTION('ref_axis',(0.,0.,-1.)) ;
#38111=DIRECTION('center_axis',(0.,0.,1.)) ;
#38112=DIRECTION('ref_axis',(1.,0.,0.)) ;
#38113=DIRECTION('center_axis',(1.,-6.12323399573679E-17,0.)) ;
#38114=DIRECTION('ref_axis',(0.,-1.,0.)) ;
#38115=DIRECTION('center_axis',(0.,0.,1.)) ;
#38116=DIRECTION('ref_axis',(1.,0.,0.)) ;
#38117=DIRECTION('center_axis',(0.,-1.22658185435577E-18,1.)) ;
#38118=DIRECTION('ref_axis',(-0.99979934733292,-0.0200316018497702,0.)) ;
#38119=DIRECTION('center_axis',(0.999353662725428,0.,-0.035947973479332)) ;
#38120=DIRECTION('ref_axis',(0.0359479734793195,0.,0.999353662725429)) ;
#38121=DIRECTION('center_axis',(0.,0.,1.)) ;
#38122=DIRECTION('ref_axis',(1.,0.,0.)) ;
#38123=DIRECTION('center_axis',(-0.999353662725428,0.,0.035947973479332)) ;
#38124=DIRECTION('ref_axis',(0.0359479734793432,0.,0.999353662725428)) ;
#38125=DIRECTION('center_axis',(0.,-0.967074537262646,-0.254493299279644)) ;
#38126=DIRECTION('ref_axis',(1.,0.,0.)) ;
#38127=DIRECTION('center_axis',(-0.999353662725428,0.,0.035947973479332)) ;
#38128=DIRECTION('ref_axis',(0.0359479734793432,0.,0.999353662725428)) ;
#38129=DIRECTION('center_axis',(0.999353662725428,0.,-0.035947973479332)) ;
#38130=DIRECTION('ref_axis',(0.035947973479332,0.,0.999353662725428)) ;
#38131=DIRECTION('',(0.999353662725428,0.,-0.035947973479332)) ;
#38132=DIRECTION('center_axis',(0.,-0.967074537262646,-0.254493299279644)) ;
#38133=DIRECTION('ref_axis',(1.,0.,0.)) ;
#38134=DIRECTION('center_axis',(0.,0.,1.)) ;
#38135=DIRECTION('ref_axis',(1.,0.,0.)) ;
#38136=DIRECTION('center_axis',(-1.22464679914737E-16,1.,0.)) ;
#38137=DIRECTION('ref_axis',(-1.,-1.22464679914737E-16,0.)) ;
#38138=DIRECTION('center_axis',(0.,0.,1.)) ;
#38139=DIRECTION('ref_axis',(1.,0.,0.)) ;
#38140=DIRECTION('center_axis',(0.,0.,-1.)) ;
#38141=DIRECTION('ref_axis',(1.,0.,0.)) ;
#38142=DIRECTION('center_axis',(0.,0.967074537262646,0.254493299279644)) ;
#38143=DIRECTION('ref_axis',(1.,-2.36847578586702E-14,-4.73695157173405E-14)) ;
#38144=DIRECTION('center_axis',(0.,0.967074537262646,0.254493299279644)) ;
#38145=DIRECTION('ref_axis',(1.,-2.36847578586702E-14,-4.73695157173405E-14)) ;
#38146=DIRECTION('center_axis',(0.,0.,-1.)) ;
#38147=DIRECTION('ref_axis',(1.,0.,0.)) ;
#38148=DIRECTION('center_axis',(0.999353662725428,0.,-0.035947973479332)) ;
#38149=DIRECTION('ref_axis',(0.035947973479332,0.,0.999353662725428)) ;
#38150=DIRECTION('center_axis',(-0.999353662725428,0.,0.035947973479332)) ;
#38151=DIRECTION('ref_axis',(0.035947973479332,0.,0.999353662725428)) ;
#38152=DIRECTION('center_axis',(0.,-0.967074537262646,-0.254493299279644)) ;
#38153=DIRECTION('ref_axis',(1.,0.,0.)) ;
#38154=DIRECTION('',(0.,-0.967074537262646,-0.254493299279644)) ;
#38155=DIRECTION('center_axis',(0.,-0.967074537262646,-0.254493299279644)) ;
#38156=DIRECTION('ref_axis',(1.,1.48029736616689E-14,4.73695157173405E-14)) ;
#38157=DIRECTION('center_axis',(0.,-0.967074537262646,-0.254493299279644)) ;
#38158=DIRECTION('ref_axis',(1.,1.48029736616689E-14,4.73695157173405E-14)) ;
#38159=DIRECTION('center_axis',(0.,0.,1.)) ;
#38160=DIRECTION('ref_axis',(1.,0.,0.)) ;
#38161=DIRECTION('center_axis',(0.,0.,1.)) ;
#38162=DIRECTION('ref_axis',(1.,0.,0.)) ;
#38163=DIRECTION('center_axis',(0.,0.,-1.)) ;
#38164=DIRECTION('ref_axis',(1.,0.,0.)) ;
#38165=DIRECTION('center_axis',(0.,0.967074537262646,0.254493299279644)) ;
#38166=DIRECTION('ref_axis',(1.,0.,0.)) ;
#38167=DIRECTION('center_axis',(0.,0.,-1.)) ;
#38168=DIRECTION('ref_axis',(1.,0.,0.)) ;
#38169=DIRECTION('center_axis',(0.,-1.,0.)) ;
#38170=DIRECTION('ref_axis',(-1.,0.,0.)) ;
#38171=DIRECTION('center_axis',(-1.,0.,0.)) ;
#38172=DIRECTION('ref_axis',(0.,-3.43024899888577E-15,-1.)) ;
#38173=DIRECTION('center_axis',(-1.,0.,0.)) ;
#38174=DIRECTION('ref_axis',(0.,0.,1.)) ;
#38175=DIRECTION('center_axis',(0.,0.,-1.)) ;
#38176=DIRECTION('ref_axis',(1.,0.,0.)) ;
#38177=DIRECTION('center_axis',(0.,0.,1.)) ;
#38178=DIRECTION('ref_axis',(1.,0.,0.)) ;
#38179=DIRECTION('',(0.,0.,-1.)) ;
#38180=DIRECTION('center_axis',(0.,0.,1.)) ;
#38181=DIRECTION('ref_axis',(1.,0.,0.)) ;
#38182=DIRECTION('center_axis',(0.,-0.967074537262646,-0.254493299279644)) ;
#38183=DIRECTION('ref_axis',(1.,0.,0.)) ;
#38184=DIRECTION('center_axis',(1.,0.,0.)) ;
#38185=DIRECTION('ref_axis',(0.,-1.,0.)) ;
#38186=DIRECTION('center_axis',(0.,0.,1.)) ;
#38187=DIRECTION('ref_axis',(1.,0.,0.)) ;
#38188=DIRECTION('center_axis',(0.,1.,0.)) ;
#38189=DIRECTION('ref_axis',(-1.,0.,0.)) ;
#47201=CARTESIAN_POINT('',(0.,0.,0.)) ;
#47202=CARTESIAN_POINT('Origin',(-57.8,19.,87.2)) ;
#47203=CARTESIAN_POINT('',(-57.8,19.,87.05)) ;
#47204=CARTESIAN_POINT('',(-57.8,19.,87.35)) ;
#47205=CARTESIAN_POINT('Origin',(-57.8,19.,87.2)) ;
#47206=CARTESIAN_POINT('Origin',(-57.8,0.,45.)) ;
#47207=CARTESIAN_POINT('',(-57.8,-1.12481983699639E-33,44.85)) ;
#47208=CARTESIAN_POINT('',(-57.8,-1.12481983699639E-33,45.15)) ;
#47209=CARTESIAN_POINT('Origin',(-57.8,0.,45.)) ;
#47210=CARTESIAN_POINT('Origin',(-20.,0.,43.6)) ;
#47211=CARTESIAN_POINT('',(-20.,-1.12481983699639E-33,43.45)) ;
#47212=CARTESIAN_POINT('',(-20.,-1.12481983699639E-33,43.75)) ;
#47213=CARTESIAN_POINT('Origin',(-20.,0.,43.6)) ;
#47214=CARTESIAN_POINT('Origin',(-20.,0.,43.6)) ;
#47215=CARTESIAN_POINT('',(-20.3765088376712,1.83697019872102E-17,43.4649404014685)) ;
#47216=CARTESIAN_POINT('Origin',(-20.3705136319189,0.,43.6148205452768)) ;
#47217=CARTESIAN_POINT('Origin',(-25.,0.,43.8)) ;
#47218=CARTESIAN_POINT('',(-29.6354815738335,-1.83697019872102E-17,43.835299310915)) ;
#47219=CARTESIAN_POINT('Origin',(-29.6294863680811,0.,43.9851794547233)) ;
#47220=CARTESIAN_POINT('',(-25.0059952057523,1.83697019872103E-17,43.6501198561917)) ;
#47221=CARTESIAN_POINT('Origin',(-30.,0.,44.)) ;
#47222=CARTESIAN_POINT('Origin',(-30.,0.,44.)) ;
#47223=CARTESIAN_POINT('',(-29.9999999999997,-0.4,44.0000000000068)) ;
#47224=CARTESIAN_POINT('',(-29.9999999999997,0.4,44.0000000000068)) ;
#47225=CARTESIAN_POINT('Origin',(-30.,0.,44.)) ;
#47226=CARTESIAN_POINT('Origin',(-30.,0.,44.)) ;
#47227=CARTESIAN_POINT('Origin',(-57.8,0.,45.)) ;
#47228=CARTESIAN_POINT('',(-57.8139063298872,0.101735781806649,44.6134040291347)) ;
#47229=CARTESIAN_POINT('',(-57.8143791893917,4.89858719658941E-17,44.6002585349098)) ;
#47230=CARTESIAN_POINT('Origin',(-57.8,0.,45.)) ;
#47231=CARTESIAN_POINT('',(-57.7860936701128,-0.101735781806649,45.3865959708653)) ;
#47232=CARTESIAN_POINT('Origin',(-57.8,0.,45.)) ;
#47233=CARTESIAN_POINT('',(-58.2,-1.06581410364015E-14,45.)) ;
#47234=CARTESIAN_POINT('Origin',(-57.8,0.,45.)) ;
#47235=CARTESIAN_POINT('Origin',(-57.8,0.,45.)) ;
#47236=CARTESIAN_POINT('Origin',(-57.8,19.,87.2)) ;
#47237=CARTESIAN_POINT('',(-57.4291900756452,18.85,87.2)) ;
#47238=CARTESIAN_POINT('',(-57.4291900756452,19.15,87.2)) ;
#47239=CARTESIAN_POINT('Origin',(-57.8,19.,87.2)) ;
#47240=CARTESIAN_POINT('Origin',(-57.4291900756452,19.,87.2)) ;
#47241=CARTESIAN_POINT('Origin',(-57.8,19.,87.2)) ;
#47242=CARTESIAN_POINT('',(-57.8,19.4,87.2)) ;
#47243=CARTESIAN_POINT('',(-58.2,19.,87.2)) ;
#47244=CARTESIAN_POINT('Origin',(-57.8,19.,87.2)) ;
#47245=CARTESIAN_POINT('',(-57.8,18.6,87.2)) ;
#47246=CARTESIAN_POINT('Origin',(-57.8,19.,87.2)) ;
#47247=CARTESIAN_POINT('Origin',(-57.8,19.,87.2)) ;
#47248=CARTESIAN_POINT('Origin',(-55.6,19.,87.2)) ;
#47249=CARTESIAN_POINT('',(-53.4,19.,87.05)) ;
#47250=CARTESIAN_POINT('Origin',(-53.4,19.,87.2)) ;
#47251=CARTESIAN_POINT('',(-57.4,19.,87.05)) ;
#47252=CARTESIAN_POINT('',(-55.6,19.,87.05)) ;
#47253=CARTESIAN_POINT('Ctrl Pts',(-57.4,19.,87.05)) ;
#47254=CARTESIAN_POINT('Ctrl Pts',(-57.4,18.9809695677553,87.05)) ;
#47255=CARTESIAN_POINT('Ctrl Pts',(-57.4014894752437,18.9607940299519,87.0538410060698)) ;
#47256=CARTESIAN_POINT('Ctrl Pts',(-57.4068656051584,18.9238876225274,87.0692083147017)) ;
#47257=CARTESIAN_POINT('Ctrl Pts',(-57.4106861522654,18.9071430958613,87.0807248697828)) ;
#47258=CARTESIAN_POINT('Ctrl Pts',(-57.4179542005944,18.8807147469091,87.1071532187349)) ;
#47259=CARTESIAN_POINT('Ctrl Pts',(-57.4218995741112,18.8692059165228,87.1238938323863)) ;
#47260=CARTESIAN_POINT('Ctrl Pts',(-57.4275680116987,18.8538444576424,87.1607852902757)) ;
#47261=CARTESIAN_POINT('Ctrl Pts',(-57.4291900756452,18.85,87.1809549836829)) ;
#47262=CARTESIAN_POINT('Ctrl Pts',(-57.4291900756452,18.85,87.2)) ;
#47263=CARTESIAN_POINT('Ctrl Pts',(-57.4291900756452,19.15,87.2)) ;
#47264=CARTESIAN_POINT('Ctrl Pts',(-57.4291900756452,19.15,87.1809549836829)) ;
#47265=CARTESIAN_POINT('Ctrl Pts',(-57.4275680116987,19.1461555423576,87.1607852902757)) ;
#47266=CARTESIAN_POINT('Ctrl Pts',(-57.4218995741112,19.1307940834772,87.1238938323863)) ;
#47267=CARTESIAN_POINT('Ctrl Pts',(-57.4179542005944,19.1192852530909,87.1071532187349)) ;
#47268=CARTESIAN_POINT('Ctrl Pts',(-57.4106861522654,19.0928569041387,87.0807248697828)) ;
#47269=CARTESIAN_POINT('Ctrl Pts',(-57.4068656051584,19.0761123774726,87.0692083147017)) ;
#47270=CARTESIAN_POINT('Ctrl Pts',(-57.4014894752437,19.0392059700481,87.0538410060698)) ;
#47271=CARTESIAN_POINT('Ctrl Pts',(-57.4,19.0190304322447,87.05)) ;
#47272=CARTESIAN_POINT('Ctrl Pts',(-57.4,19.,87.05)) ;
#47273=CARTESIAN_POINT('Origin',(-19.05,0.,43.6)) ;
#47274=CARTESIAN_POINT('',(-19.6291900756452,1.83697019872101E-17,43.75)) ;
#47275=CARTESIAN_POINT('Origin',(-19.6291900756452,0.,43.6)) ;
#47276=CARTESIAN_POINT('',(-18.1,1.83697019872103E-17,43.75)) ;
#47277=CARTESIAN_POINT('',(-19.05,-1.83697019872103E-17,43.75)) ;
#47278=CARTESIAN_POINT('Origin',(-18.1,0.,43.6)) ;
#47279=CARTESIAN_POINT('Origin',(-19.05,0.,43.6)) ;
#47280=CARTESIAN_POINT('',(-18.1,-4.89858719658941E-17,44.)) ;
#47281=CARTESIAN_POINT('Origin',(-18.1,0.,43.6)) ;
#47282=CARTESIAN_POINT('',(-19.9920031974416,-4.89858719658943E-17,44.)) ;
#47283=CARTESIAN_POINT('',(-19.05,-4.89858719658941E-17,44.)) ;
#47284=CARTESIAN_POINT('',(-20.,-0.4,43.6000000000023)) ;
#47285=CARTESIAN_POINT('Origin',(-19.9999999999996,0.,43.6)) ;
#47286=CARTESIAN_POINT('',(-20.,0.4,43.6000000000023)) ;
#47287=CARTESIAN_POINT('Origin',(-20.,0.,43.6)) ;
#47288=CARTESIAN_POINT('Origin',(-19.9999999999996,0.,43.6)) ;
#47289=CARTESIAN_POINT('Origin',(-18.1,0.,43.6)) ;
#47290=CARTESIAN_POINT('Origin',(-25.,0.,43.8)) ;
#47291=CARTESIAN_POINT('',(-20.0159872153392,4.89858719658941E-17,43.2003196165113)) ;
#47292=CARTESIAN_POINT('Origin',(-20.,0.,43.6)) ;
#47293=CARTESIAN_POINT('',(-30.0151832638221,4.8985871965894E-17,43.6002874584506)) ;
#47294=CARTESIAN_POINT('',(-25.0159872153395,4.89858719658941E-17,43.4003196165113)) ;
#47295=CARTESIAN_POINT('Origin',(-30.0000000000128,0.,44.0000000000005)) ;
#47296=CARTESIAN_POINT('Origin',(-30.0000000000128,0.,44.0000000000005)) ;
#47297=CARTESIAN_POINT('Origin',(-20.,0.,43.6)) ;
#47298=CARTESIAN_POINT('Origin',(-43.9,0.,44.5)) ;
#47299=CARTESIAN_POINT('',(-43.9143791893917,4.89858719658941E-17,44.1002585349098)) ;
#47300=CARTESIAN_POINT('Origin',(-57.8,0.,45.)) ;
#47301=CARTESIAN_POINT('Origin',(-57.8,9.5,47.5)) ;
#47302=CARTESIAN_POINT('',(-58.2,19.,50.)) ;
#47303=CARTESIAN_POINT('',(-58.2,9.5,47.5)) ;
#47304=CARTESIAN_POINT('',(-57.4,19.,50.)) ;
#47305=CARTESIAN_POINT('Origin',(-57.8,19.,50.)) ;
#47306=CARTESIAN_POINT('Origin',(-57.8,19.,50.)) ;
#47307=CARTESIAN_POINT('Origin',(-57.8,19.,68.6)) ;
#47308=CARTESIAN_POINT('Origin',(-57.8,19.,50.)) ;
#47309=CARTESIAN_POINT('',(-58.2,19.,68.6)) ;
#47310=CARTESIAN_POINT('',(-57.4,19.,86.8)) ;
#47311=CARTESIAN_POINT('Origin',(-57.8,19.,87.2)) ;
#47312=CARTESIAN_POINT('Origin',(-57.8,19.,87.2)) ;
#47313=CARTESIAN_POINT('Origin',(-57.8,19.,68.6)) ;
#47314=CARTESIAN_POINT('Origin',(-55.6,19.,87.2)) ;
#47315=CARTESIAN_POINT('',(-53.4,19.,86.8)) ;
#47316=CARTESIAN_POINT('',(-55.6,19.,86.8)) ;
#47317=CARTESIAN_POINT('Origin',(-53.4,19.,87.2)) ;
#47318=CARTESIAN_POINT('Origin',(-53.4,19.,87.2)) ;
#47319=CARTESIAN_POINT('Origin',(-57.8,19.,50.)) ;
#47320=CARTESIAN_POINT('Origin',(-20.,0.,43.6)) ;
#47321=CARTESIAN_POINT('Origin',(-20.,0.,43.6)) ;
#47322=CARTESIAN_POINT('Origin',(-30.,0.,44.)) ;
#47323=CARTESIAN_POINT('',(-30.3759624521008,1.83697019872102E-17,43.8634268159178)) ;
#47324=CARTESIAN_POINT('Origin',(-30.3705702560789,0.,44.0133298653266)) ;
#47325=CARTESIAN_POINT('Origin',(-57.8,0.,45.)) ;
#47326=CARTESIAN_POINT('',(-57.4346122660986,0.041422100489503,44.8425960181399)) ;
#47327=CARTESIAN_POINT('',(-57.434821939943,1.83697019872103E-17,44.8367670852646)) ;
#47328=CARTESIAN_POINT('Origin',(-57.4294297439211,0.,44.9866701346734)) ;
#47329=CARTESIAN_POINT('',(-57.4241851865086,-0.0348602186165462,45.1324688307429)) ;
#47330=CARTESIAN_POINT('Origin',(-57.8,0.,45.)) ;
#47331=CARTESIAN_POINT('Origin',(-57.4294297439211,0.,44.9866701346734)) ;
#47332=CARTESIAN_POINT('Origin',(-43.9,0.,44.5)) ;
#47333=CARTESIAN_POINT('',(-43.9053921960219,1.83697019872103E-17,44.3500969505912)) ;
#47334=CARTESIAN_POINT('Ctrl Pts',(-57.4346122660986,0.0414221004895022,
44.8425960181399)) ;
#47335=CARTESIAN_POINT('Ctrl Pts',(-57.4344333524598,0.0587443254615674,
44.8475698172985)) ;
#47336=CARTESIAN_POINT('Ctrl Pts',(-57.4326932970465,0.076021419458707,
44.8560347742558)) ;
#47337=CARTESIAN_POINT('Ctrl Pts',(-57.4266783464393,0.106859093622014,
44.8793548046319)) ;
#47338=CARTESIAN_POINT('Ctrl Pts',(-57.4223334613447,0.12012956463638,44.8946026069999)) ;
#47339=CARTESIAN_POINT('Ctrl Pts',(-57.414147220962,0.138975753362532,44.9266249722163)) ;
#47340=CARTESIAN_POINT('Ctrl Pts',(-57.4097459189252,0.145853589807542,
44.9456087582207)) ;
#47341=CARTESIAN_POINT('Ctrl Pts',(-57.4030911664522,0.151324256094906,
44.9849967325437)) ;
#47342=CARTESIAN_POINT('Ctrl Pts',(-57.4009030339391,0.149904658760938,
45.0054136535252)) ;
#47343=CARTESIAN_POINT('Ctrl Pts',(-57.3995805772631,0.140229844131874,
45.0421779491157)) ;
#47344=CARTESIAN_POINT('Ctrl Pts',(-57.4003662647291,0.131389448751725,
45.0607490004478)) ;
#47345=CARTESIAN_POINT('Ctrl Pts',(-57.4044547408517,0.10714444495445,45.0927035086624)) ;
#47346=CARTESIAN_POINT('Ctrl Pts',(-57.4076912940542,0.0917455512477126,
45.1060997402527)) ;
#47347=CARTESIAN_POINT('Ctrl Pts',(-57.4140390783082,0.0594496045273251,
45.1251864554143)) ;
#47348=CARTESIAN_POINT('Ctrl Pts',(-57.4175834666219,0.0403228675895078,
45.1321924635554)) ;
#47349=CARTESIAN_POINT('Ctrl Pts',(-57.4225620861009,0.00190361306705893,
45.1376824385441)) ;
#47350=CARTESIAN_POINT('Ctrl Pts',(-57.4240346154731,-0.0173306451253857,
45.1366547055289)) ;
#47351=CARTESIAN_POINT('Ctrl Pts',(-57.4241851865085,-0.0348602186165459,
45.1324688307429)) ;
#47352=CARTESIAN_POINT('Origin',(-57.8,9.5,47.5)) ;
#47353=CARTESIAN_POINT('Origin',(-30.,0.,44.)) ;
#47354=CARTESIAN_POINT('',(-30.,-1.12481983699639E-33,43.85)) ;
#47355=CARTESIAN_POINT('',(-30.,-1.12481983699639E-33,44.15)) ;
#47356=CARTESIAN_POINT('Origin',(-30.,0.,44.)) ;
#47357=CARTESIAN_POINT('Origin',(-57.8,19.,50.)) ;
#47358=CARTESIAN_POINT('',(-57.6860796798847,18.6165653110831,50.)) ;
#47359=CARTESIAN_POINT('',(-57.9139203201154,18.6165653110831,50.)) ;
#47360=CARTESIAN_POINT('Origin',(-57.8,19.,50.)) ;
#47361=CARTESIAN_POINT('',(-57.95,18.6413991639922,49.9056313589453)) ;
#47362=CARTESIAN_POINT('Origin',(-57.8,18.6413991639922,49.9056313589453)) ;
#47363=CARTESIAN_POINT('Origin',(-57.8,18.6413991639922,49.9056313589453)) ;
#47364=CARTESIAN_POINT('Origin',(-57.8,19.,68.6)) ;
#47365=CARTESIAN_POINT('Ctrl Pts',(-57.6860796798847,18.6165653110831,50.)) ;
#47366=CARTESIAN_POINT('Ctrl Pts',(-57.6886146178473,18.6158121686249,50.0028619413412)) ;
#47367=CARTESIAN_POINT('Ctrl Pts',(-57.6912408078998,18.6150594333075,50.0055921722713)) ;
#47368=CARTESIAN_POINT('Ctrl Pts',(-57.7072600366897,18.6106539924209,50.0209974725143)) ;
#47369=CARTESIAN_POINT('Ctrl Pts',(-57.7241193190454,18.6068199894771,50.0319162690223)) ;
#47370=CARTESIAN_POINT('Ctrl Pts',(-57.7610636991397,18.6014622194592,50.0463321317631)) ;
#47371=CARTESIAN_POINT('Ctrl Pts',(-57.7811519935343,18.6,50.0498438108241)) ;
#47372=CARTESIAN_POINT('Ctrl Pts',(-57.8188480064657,18.6,50.0498438108241)) ;
#47373=CARTESIAN_POINT('Ctrl Pts',(-57.8389363008603,18.6014622194592,50.0463321317631)) ;
#47374=CARTESIAN_POINT('Ctrl Pts',(-57.8758806809546,18.6068199894771,50.0319162690223)) ;
#47375=CARTESIAN_POINT('Ctrl Pts',(-57.8927399633103,18.6106539924209,50.0209974725143)) ;
#47376=CARTESIAN_POINT('Ctrl Pts',(-57.9087591921002,18.6150594333075,50.0055921722713)) ;
#47377=CARTESIAN_POINT('Ctrl Pts',(-57.9113853821527,18.6158121686249,50.0028619413412)) ;
#47378=CARTESIAN_POINT('Ctrl Pts',(-57.9139203201154,18.6165653110831,50.)) ;
#47379=CARTESIAN_POINT('Origin',(-43.9,0.,44.5)) ;
#47380=CARTESIAN_POINT('',(-57.8018230872335,0.396772011309262,44.9493181749091)) ;
#47381=CARTESIAN_POINT('',(-57.7913960076435,0.320489692203214,45.2391909875121)) ;
#47382=CARTESIAN_POINT('Ctrl Pts',(-57.8018230872335,0.396772011309261,
44.9493181749091)) ;
#47383=CARTESIAN_POINT('Ctrl Pts',(-57.7838099638155,0.396827731634953,
44.9491064376715)) ;
#47384=CARTESIAN_POINT('Ctrl Pts',(-57.7648197232592,0.397403006824304,
44.9525521245349)) ;
#47385=CARTESIAN_POINT('Ctrl Pts',(-57.7285306259727,0.398930598445194,
44.9670570197925)) ;
#47386=CARTESIAN_POINT('Ctrl Pts',(-57.7113958074383,0.399819549885464,
44.9785768936597)) ;
#47387=CARTESIAN_POINT('Ctrl Pts',(-57.6840433857854,0.400129413279351,
45.0050225681604)) ;
#47388=CARTESIAN_POINT('Ctrl Pts',(-57.6719414680996,0.399565898583832,
45.0217756379422)) ;
#47389=CARTESIAN_POINT('Ctrl Pts',(-57.655291417997,0.395377554048088,45.0582755050382)) ;
#47390=CARTESIAN_POINT('Ctrl Pts',(-57.650752206554,0.391685614070328,45.078018639465)) ;
#47391=CARTESIAN_POINT('Ctrl Pts',(-57.6494291476468,0.382006393643826,
45.1147996770857)) ;
#47392=CARTESIAN_POINT('Ctrl Pts',(-57.6525653247154,0.375434029513804,
45.1340608982685)) ;
#47393=CARTESIAN_POINT('Ctrl Pts',(-57.6666482059757,0.360841507256248,
45.168928324987)) ;
#47394=CARTESIAN_POINT('Ctrl Pts',(-57.6775850700919,0.352881735310964,
45.1845637444403)) ;
#47395=CARTESIAN_POINT('Ctrl Pts',(-57.7030996592059,0.33912667597473,45.2092098145205)) ;
#47396=CARTESIAN_POINT('Ctrl Pts',(-57.7194346236979,0.332386160750563,
45.2199258830321)) ;
#47397=CARTESIAN_POINT('Ctrl Pts',(-57.754688260616,0.323283359066371,45.234206786015)) ;
#47398=CARTESIAN_POINT('Ctrl Pts',(-57.7734112133181,0.320752662206818,
45.2381917014984)) ;
#47399=CARTESIAN_POINT('Ctrl Pts',(-57.7913960076435,0.320489692203213,
45.2391909875121)) ;
#47400=CARTESIAN_POINT('Origin',(-57.8,0.,45.)) ;
#47401=CARTESIAN_POINT('Origin',(-57.8,9.5,47.5)) ;
#47402=CARTESIAN_POINT('',(-57.95,0.358600836007785,45.0943686410547)) ;
#47403=CARTESIAN_POINT('',(-57.95,9.5,47.5)) ;
#47404=CARTESIAN_POINT('Origin',(-57.8,0.358600836007795,45.0943686410547)) ;
#47405=CARTESIAN_POINT('Origin',(-57.8,0.358600836007795,45.0943686410547)) ;
#47406=CARTESIAN_POINT('Origin',(-57.8,0.,45.)) ;
#47407=CARTESIAN_POINT('Origin',(-57.8,19.,50.)) ;
#47408=CARTESIAN_POINT('',(-57.9139203201153,18.9024184409593,50.3708099243548)) ;
#47409=CARTESIAN_POINT('',(-57.95,19.,50.3708099243548)) ;
#47410=CARTESIAN_POINT('Origin',(-57.8,19.,50.3708099243548)) ;
#47411=CARTESIAN_POINT('',(-57.6860796798847,18.9024184409593,50.3708099243548)) ;
#47412=CARTESIAN_POINT('Origin',(-57.8,19.,50.)) ;
#47413=CARTESIAN_POINT('Origin',(-57.8,19.,50.3708099243548)) ;
#47414=CARTESIAN_POINT('',(-57.8,19.,50.4)) ;
#47415=CARTESIAN_POINT('Origin',(-57.8,19.,50.)) ;
#47416=CARTESIAN_POINT('Origin',(-55.6,19.,87.2)) ;
#47417=CARTESIAN_POINT('',(-57.8,19.15,86.8291900756452)) ;
#47418=CARTESIAN_POINT('',(-57.8,18.85,86.8291900756452)) ;
#47419=CARTESIAN_POINT('Ctrl Pts',(-57.8,19.15,86.8291900756452)) ;
#47420=CARTESIAN_POINT('Ctrl Pts',(-57.7809549836829,19.15,86.8291900756452)) ;
#47421=CARTESIAN_POINT('Ctrl Pts',(-57.7607852902757,19.1461555423576,86.8275680116987)) ;
#47422=CARTESIAN_POINT('Ctrl Pts',(-57.7238938323863,19.1307940834772,86.8218995741112)) ;
#47423=CARTESIAN_POINT('Ctrl Pts',(-57.7071532187349,19.1192852530909,86.8179542005944)) ;
#47424=CARTESIAN_POINT('Ctrl Pts',(-57.6807248697828,19.0928569041387,86.8106861522654)) ;
#47425=CARTESIAN_POINT('Ctrl Pts',(-57.6692083147017,19.0761123774726,86.8068656051584)) ;
#47426=CARTESIAN_POINT('Ctrl Pts',(-57.6538410060698,19.0392059700481,86.8014894752437)) ;
#47427=CARTESIAN_POINT('Ctrl Pts',(-57.65,19.0190304322447,86.8)) ;
#47428=CARTESIAN_POINT('Ctrl Pts',(-57.65,18.9809695677553,86.8)) ;
#47429=CARTESIAN_POINT('Ctrl Pts',(-57.6538410060698,18.9607940299519,86.8014894752437)) ;
#47430=CARTESIAN_POINT('Ctrl Pts',(-57.6692083147017,18.9238876225274,86.8068656051584)) ;
#47431=CARTESIAN_POINT('Ctrl Pts',(-57.6807248697828,18.9071430958613,86.8106861522654)) ;
#47432=CARTESIAN_POINT('Ctrl Pts',(-57.7071532187349,18.8807147469091,86.8179542005944)) ;
#47433=CARTESIAN_POINT('Ctrl Pts',(-57.7238938323863,18.8692059165228,86.8218995741112)) ;
#47434=CARTESIAN_POINT('Ctrl Pts',(-57.7607852902757,18.8538444576424,86.8275680116987)) ;
#47435=CARTESIAN_POINT('Ctrl Pts',(-57.7809549836829,18.85,86.8291900756452)) ;
#47436=CARTESIAN_POINT('Ctrl Pts',(-57.8,18.85,86.8291900756452)) ;
#47437=CARTESIAN_POINT('Origin',(-57.8,19.,87.2)) ;
#47438=CARTESIAN_POINT('Origin',(-57.8,19.,68.6)) ;
#47439=CARTESIAN_POINT('',(-57.95,19.,86.8291900756452)) ;
#47440=CARTESIAN_POINT('Origin',(-57.8,19.,86.8291900756452)) ;
#47441=CARTESIAN_POINT('',(-57.95,19.,68.6)) ;
#47442=CARTESIAN_POINT('Ctrl Pts',(-57.6860796798847,18.9024184409593,50.3708099243548)) ;
#47443=CARTESIAN_POINT('Ctrl Pts',(-57.6885032122124,18.8995891197094,50.3708099243548)) ;
#47444=CARTESIAN_POINT('Ctrl Pts',(-57.6910096124592,18.8968769056013,50.3708402030569)) ;
#47445=CARTESIAN_POINT('Ctrl Pts',(-57.7069183737083,18.8808606548532,50.3711657794823)) ;
#47446=CARTESIAN_POINT('Ctrl Pts',(-57.7238219217715,18.869232921536,50.3720978089255)) ;
#47447=CARTESIAN_POINT('Ctrl Pts',(-57.7608947554465,18.853801818028,50.3736194963427)) ;
#47448=CARTESIAN_POINT('Ctrl Pts',(-57.7810672966117,18.85,50.3741448990397)) ;
#47449=CARTESIAN_POINT('Ctrl Pts',(-57.8189327033883,18.85,50.3741448990398)) ;
#47450=CARTESIAN_POINT('Ctrl Pts',(-57.8391052445535,18.853801818028,50.3736194963427)) ;
#47451=CARTESIAN_POINT('Ctrl Pts',(-57.8761780782285,18.869232921536,50.3720978089255)) ;
#47452=CARTESIAN_POINT('Ctrl Pts',(-57.8930816262917,18.8808606548532,50.3711657794824)) ;
#47453=CARTESIAN_POINT('Ctrl Pts',(-57.9089903875408,18.8968769056013,50.3708402030569)) ;
#47454=CARTESIAN_POINT('Ctrl Pts',(-57.9114967877876,18.8995891197094,50.3708099243548)) ;
#47455=CARTESIAN_POINT('Ctrl Pts',(-57.9139203201153,18.9024184409593,50.3708099243548)) ;
#47456=CARTESIAN_POINT('Origin',(-57.8,19.,86.8291900756452)) ;
#47457=CARTESIAN_POINT('Origin',(-57.8,9.5,47.5)) ;
#47458=CARTESIAN_POINT('Origin',(-57.8,19.,87.2)) ;
#47459=CARTESIAN_POINT('Origin',(-57.8,19.,50.)) ;
#47460=CARTESIAN_POINT('',(-57.8,19.,49.85)) ;
#47461=CARTESIAN_POINT('',(-57.8,19.,50.15)) ;
#47462=CARTESIAN_POINT('Origin',(-57.8,19.,50.)) ;
#50368=UNCERTAINTY_MEASURE_WITH_UNIT(LENGTH_MEASURE(0.001),#50441,
'DISTANCE_ACCURACY_VALUE',
'Maximum model space distance between geometric entities at asserted c
onnectivities') ;
#50387=UNCERTAINTY_MEASURE_WITH_UNIT(LENGTH_MEASURE(0.001),#50441,
'DISTANCE_ACCURACY_VALUE',
'Maximum model space distance between geometric entities at asserted c
onnectivities') ;
#50421=(
GEOMETRIC_REPRESENTATION_CONTEXT(3)
GLOBAL_UNCERTAINTY_ASSIGNED_CONTEXT((#50368))
GLOBAL_UNIT_ASSIGNED_CONTEXT((#50441,#50443,#50444))
REPRESENTATION_CONTEXT('','3D')
) ;
#50440=(
GEOMETRIC_REPRESENTATION_CONTEXT(3)
GLOBAL_UNCERTAINTY_ASSIGNED_CONTEXT((#50387))
GLOBAL_UNIT_ASSIGNED_CONTEXT((#50441,#50443,#50444))
REPRESENTATION_CONTEXT('','3D')
) ;
#50441=(
LENGTH_UNIT()
NAMED_UNIT(*)
SI_UNIT(.CENTI.,.METRE.)
) ;
#50443=(
NAMED_UNIT(*)
PLANE_ANGLE_UNIT()
SI_UNIT($,.RADIAN.)
) ;
#50444=(
NAMED_UNIT(*)
SI_UNIT($,.STERADIAN.)
SOLID_ANGLE_UNIT()
) ;
#50478=SHAPE_DEFINITION_REPRESENTATION(#50554,#50652) ;
#50554=PRODUCT_DEFINITION_SHAPE('',$,#50705) ;
#50652=SHAPE_REPRESENTATION('',(#30942),#50421) ;
#50671=PRODUCT_DEFINITION_CONTEXT('part definition',#50829,'design') ;
#50705=PRODUCT_DEFINITION('CONTROL_CABLE_SHEATH',
'CONTROL_CABLE_SHEATH',#50757,#50671) ;
#50757=PRODUCT_DEFINITION_FORMATION('',$,#50864) ;
#50829=APPLICATION_CONTEXT(
'Core Data for Automotive Mechanical Design Process') ;
#50830=PRODUCT_CONTEXT('part definition',#50829,'mechanical') ;
#50864=PRODUCT('CONTROL_CABLE_SHEATH','CONTROL_CABLE_SHEATH',$,(#50830)) ;
#50888=PRESENTATION_STYLE_ASSIGNMENT((#50895)) ;
#50895=SURFACE_STYLE_USAGE(.BOTH.,#50902) ;
#50902=SURFACE_SIDE_STYLE('',(#50909)) ;
#50909=SURFACE_STYLE_FILL_AREA(#50916) ;
#50916=FILL_AREA_STYLE('Rubber - Soft',(#50923)) ;
#50923=FILL_AREA_STYLE_COLOUR('Rubber - Soft',#50930) ;
#50930=COLOUR_RGB('Rubber - Soft', 0.40784314, 0.44705882, 0.49803922) ;
ENDSEC;
END-ISO-10303-21;
